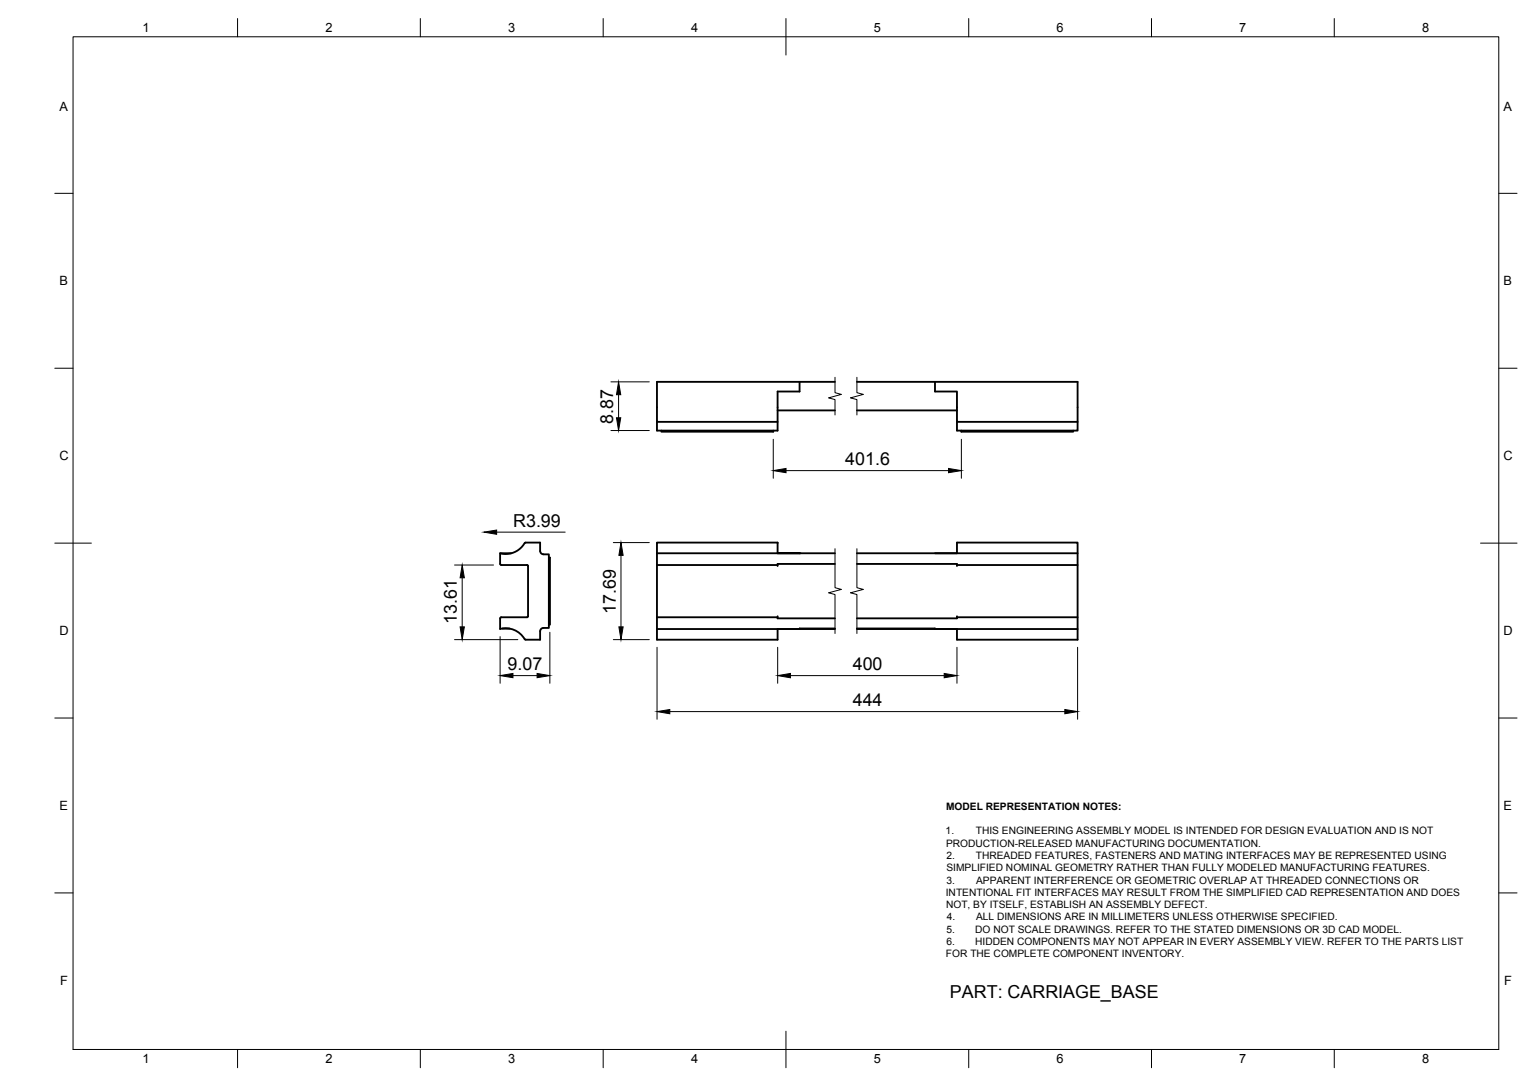
ISO-10303-21;
HEADER;
/* Generated by software containing ST-Developer
 * from STEP Tools, Inc. (www.steptools.com) 
 */

FILE_DESCRIPTION(
/* description */ (''),
/* implementation_level */ '2;1');

FILE_NAME(
/* name */ 'Carriage_Base.step',
/* time_stamp */ '2026-10-05T11:01:41-07:00',
/* author */ (''),
/* organization */ (''),
/* preprocessor_version */ 'ST-DEVELOPER v20.2',
/* originating_system */ 'Autodesk Translation Framework v15.15.0.0',
/* authorisation */ '');

FILE_SCHEMA (('AUTOMOTIVE_DESIGN { 1 0 10303 214 3 1 1 }'));
ENDSEC;

DATA;
#10=MECHANICAL_DESIGN_GEOMETRIC_PRESENTATION_REPRESENTATION('',(#2143),#215609);
#216=FACE_BOUND('',#5119,.T.);
#217=FACE_BOUND('',#5154,.T.);
#2125=SHAPE_REPRESENTATION_RELATIONSHIP('SRR','None',#215650,#2134);
#2134=ADVANCED_BREP_SHAPE_REPRESENTATION('',(#2152),#215606);
#2143=STYLED_ITEM('',(#215698),#2152);
#2152=MANIFOLD_SOLID_BREP('Body1',#28086);
#2632=CYLINDRICAL_SURFACE('',#29448,0.190999999999998);
#2633=CYLINDRICAL_SURFACE('',#29461,0.191);
#2634=CYLINDRICAL_SURFACE('',#29467,3.9858295958384);
#2635=CYLINDRICAL_SURFACE('',#29468,3.9858295958384);
#2636=CYLINDRICAL_SURFACE('',#29480,0.190999999999999);
#2637=CYLINDRICAL_SURFACE('',#29482,0.191);
#2638=CYLINDRICAL_SURFACE('',#29483,0.590999999999999);
#2639=CYLINDRICAL_SURFACE('',#29484,0.590999999999999);
#2640=CYLINDRICAL_SURFACE('',#29485,0.191000000000001);
#2641=CYLINDRICAL_SURFACE('',#29487,0.190999999999999);
#2642=CYLINDRICAL_SURFACE('',#29504,0.190999999999998);
#2643=CYLINDRICAL_SURFACE('',#29518,0.191);
#2644=CYLINDRICAL_SURFACE('',#29524,3.9858295958384);
#2645=CYLINDRICAL_SURFACE('',#29525,3.9858295958384);
#2646=CYLINDRICAL_SURFACE('',#29542,0.190999999999999);
#2647=CYLINDRICAL_SURFACE('',#29544,0.191);
#2648=CYLINDRICAL_SURFACE('',#29545,0.590999999999999);
#2649=CYLINDRICAL_SURFACE('',#29546,0.590999999999999);
#2650=CYLINDRICAL_SURFACE('',#29547,0.191000000000001);
#2651=CYLINDRICAL_SURFACE('',#29549,0.190999999999999);
#3752=FACE_OUTER_BOUND('',#5108,.T.);
#3753=FACE_OUTER_BOUND('',#5109,.T.);
#3754=FACE_OUTER_BOUND('',#5110,.T.);
#3755=FACE_OUTER_BOUND('',#5111,.T.);
#3756=FACE_OUTER_BOUND('',#5112,.T.);
#3757=FACE_OUTER_BOUND('',#5113,.T.);
#3758=FACE_OUTER_BOUND('',#5114,.T.);
#3759=FACE_OUTER_BOUND('',#5115,.T.);
#3760=FACE_OUTER_BOUND('',#5116,.T.);
#3761=FACE_OUTER_BOUND('',#5117,.T.);
#3762=FACE_OUTER_BOUND('',#5118,.T.);
#3763=FACE_OUTER_BOUND('',#5120,.T.);
#3764=FACE_OUTER_BOUND('',#5121,.T.);
#3765=FACE_OUTER_BOUND('',#5122,.T.);
#3766=FACE_OUTER_BOUND('',#5123,.T.);
#3767=FACE_OUTER_BOUND('',#5124,.T.);
#3768=FACE_OUTER_BOUND('',#5125,.T.);
#3769=FACE_OUTER_BOUND('',#5126,.T.);
#3770=FACE_OUTER_BOUND('',#5127,.T.);
#3771=FACE_OUTER_BOUND('',#5128,.T.);
#3772=FACE_OUTER_BOUND('',#5129,.T.);
#3773=FACE_OUTER_BOUND('',#5130,.T.);
#3774=FACE_OUTER_BOUND('',#5131,.T.);
#3775=FACE_OUTER_BOUND('',#5132,.T.);
#3776=FACE_OUTER_BOUND('',#5133,.T.);
#3777=FACE_OUTER_BOUND('',#5134,.T.);
#3778=FACE_OUTER_BOUND('',#5135,.T.);
#3779=FACE_OUTER_BOUND('',#5136,.T.);
#3780=FACE_OUTER_BOUND('',#5137,.T.);
#3781=FACE_OUTER_BOUND('',#5138,.T.);
#3782=FACE_OUTER_BOUND('',#5139,.T.);
#3783=FACE_OUTER_BOUND('',#5140,.T.);
#3784=FACE_OUTER_BOUND('',#5141,.T.);
#3785=FACE_OUTER_BOUND('',#5142,.T.);
#3786=FACE_OUTER_BOUND('',#5143,.T.);
#3787=FACE_OUTER_BOUND('',#5144,.T.);
#3788=FACE_OUTER_BOUND('',#5145,.T.);
#3789=FACE_OUTER_BOUND('',#5146,.T.);
#3790=FACE_OUTER_BOUND('',#5147,.T.);
#3791=FACE_OUTER_BOUND('',#5148,.T.);
#3792=FACE_OUTER_BOUND('',#5149,.T.);
#3793=FACE_OUTER_BOUND('',#5150,.T.);
#3794=FACE_OUTER_BOUND('',#5151,.T.);
#3795=FACE_OUTER_BOUND('',#5152,.T.);
#3796=FACE_OUTER_BOUND('',#5153,.T.);
#3797=FACE_OUTER_BOUND('',#5155,.T.);
#3798=FACE_OUTER_BOUND('',#5156,.T.);
#3799=FACE_OUTER_BOUND('',#5157,.T.);
#3800=FACE_OUTER_BOUND('',#5158,.T.);
#3801=FACE_OUTER_BOUND('',#5159,.T.);
#3802=FACE_OUTER_BOUND('',#5160,.T.);
#3803=FACE_OUTER_BOUND('',#5161,.T.);
#3804=FACE_OUTER_BOUND('',#5162,.T.);
#3805=FACE_OUTER_BOUND('',#5163,.T.);
#3806=FACE_OUTER_BOUND('',#5164,.T.);
#3807=FACE_OUTER_BOUND('',#5165,.T.);
#3808=FACE_OUTER_BOUND('',#5166,.T.);
#3809=FACE_OUTER_BOUND('',#5167,.T.);
#3810=FACE_OUTER_BOUND('',#5168,.T.);
#3811=FACE_OUTER_BOUND('',#5169,.T.);
#3812=FACE_OUTER_BOUND('',#5170,.T.);
#3813=FACE_OUTER_BOUND('',#5171,.T.);
#3814=FACE_OUTER_BOUND('',#5172,.T.);
#3815=FACE_OUTER_BOUND('',#5173,.T.);
#3816=FACE_OUTER_BOUND('',#5174,.T.);
#3817=FACE_OUTER_BOUND('',#5175,.T.);
#3818=FACE_OUTER_BOUND('',#5176,.T.);
#3819=FACE_OUTER_BOUND('',#5177,.T.);
#3820=FACE_OUTER_BOUND('',#5178,.T.);
#3821=FACE_OUTER_BOUND('',#5179,.T.);
#5108=EDGE_LOOP('',(#22607,#22608,#22609));
#5109=EDGE_LOOP('',(#22610,#22611,#22612));
#5110=EDGE_LOOP('',(#22613,#22614));
#5111=EDGE_LOOP('',(#22615,#22616,#22617,#22618));
#5112=EDGE_LOOP('',(#22619,#22620,#22621,#22622,#22623,#22624,#22625,#22626,
#22627,#22628,#22629,#22630,#22631,#22632,#22633,#22634));
#5113=EDGE_LOOP('',(#22635,#22636,#22637,#22638));
#5114=EDGE_LOOP('',(#22639,#22640,#22641,#22642));
#5115=EDGE_LOOP('',(#22643,#22644,#22645,#22646,#22647,#22648,#22649,#22650,
#22651,#22652,#22653,#22654,#22655,#22656,#22657,#22658,#22659,#22660,#22661,
#22662,#22663,#22664));
#5116=EDGE_LOOP('',(#22665,#22666,#22667,#22668));
#5117=EDGE_LOOP('',(#22669,#22670,#22671,#22672));
#5118=EDGE_LOOP('',(#22673,#22674,#22675,#22676));
#5119=EDGE_LOOP('',(#22677,#22678,#22679,#22680));
#5120=EDGE_LOOP('',(#22681,#22682,#22683,#22684));
#5121=EDGE_LOOP('',(#22685,#22686,#22687,#22688));
#5122=EDGE_LOOP('',(#22689,#22690,#22691,#22692));
#5123=EDGE_LOOP('',(#22693,#22694,#22695,#22696,#22697,#22698));
#5124=EDGE_LOOP('',(#22699,#22700,#22701,#22702,#22703,#22704,#22705));
#5125=EDGE_LOOP('',(#22706,#22707,#22708,#22709));
#5126=EDGE_LOOP('',(#22710,#22711,#22712,#22713));
#5127=EDGE_LOOP('',(#22714,#22715,#22716,#22717));
#5128=EDGE_LOOP('',(#22718,#22719,#22720,#22721));
#5129=EDGE_LOOP('',(#22722,#22723,#22724,#22725));
#5130=EDGE_LOOP('',(#22726,#22727,#22728,#22729,#22730));
#5131=EDGE_LOOP('',(#22731,#22732,#22733,#22734,#22735));
#5132=EDGE_LOOP('',(#22736,#22737,#22738,#22739));
#5133=EDGE_LOOP('',(#22740,#22741,#22742,#22743));
#5134=EDGE_LOOP('',(#22744,#22745,#22746,#22747));
#5135=EDGE_LOOP('',(#22748,#22749,#22750,#22751));
#5136=EDGE_LOOP('',(#22752,#22753,#22754,#22755));
#5137=EDGE_LOOP('',(#22756,#22757,#22758,#22759));
#5138=EDGE_LOOP('',(#22760,#22761,#22762,#22763));
#5139=EDGE_LOOP('',(#22764,#22765,#22766,#22767));
#5140=EDGE_LOOP('',(#22768,#22769,#22770));
#5141=EDGE_LOOP('',(#22771,#22772,#22773));
#5142=EDGE_LOOP('',(#22774,#22775));
#5143=EDGE_LOOP('',(#22776,#22777,#22778,#22779,#22780,#22781,#22782,#22783));
#5144=EDGE_LOOP('',(#22784,#22785,#22786,#22787));
#5145=EDGE_LOOP('',(#22788,#22789,#22790,#22791,#22792,#22793,#22794,#22795,
#22796,#22797,#22798,#22799,#22800,#22801,#22802,#22803));
#5146=EDGE_LOOP('',(#22804,#22805,#22806,#22807,#22808,#22809,#22810,#22811,
#22812,#22813));
#5147=EDGE_LOOP('',(#22814,#22815,#22816,#22817));
#5148=EDGE_LOOP('',(#22818,#22819,#22820,#22821));
#5149=EDGE_LOOP('',(#22822,#22823,#22824,#22825,#22826,#22827,#22828,#22829,
#22830,#22831,#22832,#22833,#22834,#22835,#22836,#22837,#22838,#22839,#22840,
#22841,#22842,#22843));
#5150=EDGE_LOOP('',(#22844,#22845,#22846,#22847,#22848,#22849,#22850,#22851,
#22852,#22853));
#5151=EDGE_LOOP('',(#22854,#22855,#22856,#22857));
#5152=EDGE_LOOP('',(#22858,#22859,#22860,#22861));
#5153=EDGE_LOOP('',(#22862,#22863,#22864,#22865));
#5154=EDGE_LOOP('',(#22866,#22867,#22868,#22869));
#5155=EDGE_LOOP('',(#22870,#22871,#22872,#22873));
#5156=EDGE_LOOP('',(#22874,#22875,#22876,#22877));
#5157=EDGE_LOOP('',(#22878,#22879,#22880,#22881));
#5158=EDGE_LOOP('',(#22882,#22883,#22884,#22885,#22886,#22887));
#5159=EDGE_LOOP('',(#22888,#22889,#22890,#22891,#22892,#22893,#22894));
#5160=EDGE_LOOP('',(#22895,#22896,#22897,#22898));
#5161=EDGE_LOOP('',(#22899,#22900,#22901,#22902));
#5162=EDGE_LOOP('',(#22903,#22904,#22905,#22906));
#5163=EDGE_LOOP('',(#22907,#22908,#22909,#22910));
#5164=EDGE_LOOP('',(#22911,#22912,#22913,#22914));
#5165=EDGE_LOOP('',(#22915,#22916,#22917,#22918));
#5166=EDGE_LOOP('',(#22919,#22920,#22921,#22922));
#5167=EDGE_LOOP('',(#22923,#22924,#22925,#22926));
#5168=EDGE_LOOP('',(#22927,#22928,#22929,#22930,#22931));
#5169=EDGE_LOOP('',(#22932,#22933,#22934,#22935,#22936));
#5170=EDGE_LOOP('',(#22937,#22938,#22939,#22940,#22941,#22942,#22943,#22944,
#22945,#22946));
#5171=EDGE_LOOP('',(#22947,#22948,#22949,#22950,#22951,#22952,#22953,#22954,
#22955,#22956,#22957,#22958));
#5172=EDGE_LOOP('',(#22959,#22960,#22961,#22962));
#5173=EDGE_LOOP('',(#22963,#22964,#22965,#22966));
#5174=EDGE_LOOP('',(#22967,#22968,#22969,#22970));
#5175=EDGE_LOOP('',(#22971,#22972,#22973,#22974));
#5176=EDGE_LOOP('',(#22975,#22976,#22977,#22978));
#5177=EDGE_LOOP('',(#22979,#22980,#22981,#22982));
#5178=EDGE_LOOP('',(#22983,#22984,#22985,#22986));
#5179=EDGE_LOOP('',(#22987,#22988,#22989,#22990));
#6088=CIRCLE('',#29435,3.9858295958384);
#6089=CIRCLE('',#29437,3.9858295958384);
#6090=CIRCLE('',#29439,3.9858295958384);
#6091=CIRCLE('',#29442,3.9858295958384);
#6092=CIRCLE('',#29443,3.9858295958384);
#6093=CIRCLE('',#29444,0.191);
#6094=CIRCLE('',#29445,0.590999999999999);
#6095=CIRCLE('',#29446,0.590999999999999);
#6096=CIRCLE('',#29447,0.190999999999998);
#6097=CIRCLE('',#29449,0.190999999999998);
#6098=CIRCLE('',#29452,0.590999999999999);
#6099=CIRCLE('',#29453,0.590999999999999);
#6100=CIRCLE('',#29454,0.191);
#6101=CIRCLE('',#29455,3.9858295958384);
#6102=CIRCLE('',#29456,0.191000000000001);
#6103=CIRCLE('',#29457,0.190999999999999);
#6104=CIRCLE('',#29458,0.190999999999999);
#6105=CIRCLE('',#29459,0.191);
#6106=CIRCLE('',#29460,3.9858295958384);
#6107=CIRCLE('',#29475,0.191);
#6108=CIRCLE('',#29476,0.190999999999999);
#6109=CIRCLE('',#29478,0.190999999999999);
#6110=CIRCLE('',#29479,0.191000000000001);
#6111=CIRCLE('',#29489,3.9858295958384);
#6112=CIRCLE('',#29491,3.9858295958384);
#6113=CIRCLE('',#29493,3.9858295958384);
#6114=CIRCLE('',#29497,3.9858295958384);
#6115=CIRCLE('',#29498,0.190999999999998);
#6116=CIRCLE('',#29499,0.590999999999999);
#6117=CIRCLE('',#29500,0.590999999999999);
#6118=CIRCLE('',#29501,0.191);
#6119=CIRCLE('',#29502,3.9858295958384);
#6120=CIRCLE('',#29505,0.190999999999998);
#6121=CIRCLE('',#29508,3.9858295958384);
#6122=CIRCLE('',#29509,0.191);
#6123=CIRCLE('',#29510,0.190999999999999);
#6124=CIRCLE('',#29511,0.190999999999999);
#6125=CIRCLE('',#29512,0.191000000000001);
#6126=CIRCLE('',#29513,3.9858295958384);
#6127=CIRCLE('',#29514,0.191);
#6128=CIRCLE('',#29515,0.590999999999999);
#6129=CIRCLE('',#29516,0.590999999999999);
#6130=CIRCLE('',#29535,0.190999999999999);
#6131=CIRCLE('',#29536,0.191);
#6132=CIRCLE('',#29538,0.191000000000001);
#6133=CIRCLE('',#29539,0.190999999999999);
#7371=LINE('',#127456,#9216);
#7372=LINE('',#127458,#9217);
#7373=LINE('',#127463,#9218);
#7374=LINE('',#127466,#9219);
#7375=LINE('',#127470,#9220);
#7376=LINE('',#127474,#9221);
#7377=LINE('',#127476,#9222);
#7378=LINE('',#127478,#9223);
#7379=LINE('',#127479,#9224);
#7380=LINE('',#127485,#9225);
#7381=LINE('',#127487,#9226);
#7382=LINE('',#127489,#9227);
#7383=LINE('',#127494,#9228);
#7384=LINE('',#127498,#9229);
#7385=LINE('',#127500,#9230);
#7386=LINE('',#127502,#9231);
#7387=LINE('',#127506,#9232);
#7388=LINE('',#127508,#9233);
#7389=LINE('',#127514,#9234);
#7390=LINE('',#127515,#9235);
#7391=LINE('',#127518,#9236);
#7392=LINE('',#127519,#9237);
#7393=LINE('',#127522,#9238);
#7394=LINE('',#127526,#9239);
#7395=LINE('',#127528,#9240);
#7396=LINE('',#127530,#9241);
#7397=LINE('',#127533,#9242);
#7398=LINE('',#127539,#9243);
#7399=LINE('',#127543,#9244);
#7400=LINE('',#127547,#9245);
#7401=LINE('',#127551,#9246);
#7402=LINE('',#127555,#9247);
#7403=LINE('',#127558,#9248);
#7404=LINE('',#127560,#9249);
#7405=LINE('',#127562,#9250);
#7406=LINE('',#127563,#9251);
#7407=LINE('',#127566,#9252);
#7408=LINE('',#127568,#9253);
#7409=LINE('',#127570,#9254);
#7410=LINE('',#127571,#9255);
#7411=LINE('',#127573,#9256);
#7412=LINE('',#127575,#9257);
#7413=LINE('',#127577,#9258);
#7414=LINE('',#127579,#9259);
#7415=LINE('',#127580,#9260);
#7416=LINE('',#127582,#9261);
#7417=LINE('',#127583,#9262);
#7418=LINE('',#127586,#9263);
#7419=LINE('',#127588,#9264);
#7420=LINE('',#127589,#9265);
#7421=LINE('',#127592,#9266);
#7422=LINE('',#127593,#9267);
#7423=LINE('',#127596,#9268);
#7424=LINE('',#127597,#9269);
#7425=LINE('',#127599,#9270);
#7426=LINE('',#127604,#9271);
#7427=LINE('',#127608,#9272);
#7428=LINE('',#127611,#9273);
#7429=LINE('',#127615,#9274);
#7430=LINE('',#127617,#9275);
#7431=LINE('',#127621,#9276);
#7432=LINE('',#127624,#9277);
#7433=LINE('',#127625,#9278);
#7434=LINE('',#127627,#9279);
#7435=LINE('',#127629,#9280);
#7436=LINE('',#127633,#9281);
#7437=LINE('',#127634,#9282);
#7438=LINE('',#127636,#9283);
#7439=LINE('',#127638,#9284);
#7440=LINE('',#127642,#9285);
#7441=LINE('',#127645,#9286);
#7442=LINE('',#127649,#9287);
#7443=LINE('',#127651,#9288);
#7444=LINE('',#127656,#9289);
#7445=LINE('',#127659,#9290);
#7446=LINE('',#127661,#9291);
#7447=LINE('',#127662,#9292);
#7448=LINE('',#127663,#9293);
#7449=LINE('',#127667,#9294);
#7450=LINE('',#127669,#9295);
#7451=LINE('',#127671,#9296);
#7452=LINE('',#127672,#9297);
#7453=LINE('',#127679,#9298);
#7454=LINE('',#127681,#9299);
#7455=LINE('',#127685,#9300);
#7456=LINE('',#127687,#9301);
#7457=LINE('',#127689,#9302);
#7458=LINE('',#127692,#9303);
#7459=LINE('',#127698,#9304);
#7460=LINE('',#127699,#9305);
#7461=LINE('',#127701,#9306);
#7462=LINE('',#127702,#9307);
#7463=LINE('',#127703,#9308);
#7464=LINE('',#127708,#9309);
#7465=LINE('',#127709,#9310);
#7466=LINE('',#127712,#9311);
#7467=LINE('',#127713,#9312);
#7468=LINE('',#127718,#9313);
#7469=LINE('',#127722,#9314);
#7470=LINE('',#127726,#9315);
#7471=LINE('',#127730,#9316);
#7472=LINE('',#127734,#9317);
#7473=LINE('',#127739,#9318);
#7474=LINE('',#127743,#9319);
#7475=LINE('',#127745,#9320);
#7476=LINE('',#127747,#9321);
#7477=LINE('',#127750,#9322);
#7478=LINE('',#127753,#9323);
#7479=LINE('',#127754,#9324);
#7480=LINE('',#127755,#9325);
#7481=LINE('',#127757,#9326);
#7482=LINE('',#127759,#9327);
#7483=LINE('',#127761,#9328);
#7484=LINE('',#127762,#9329);
#7485=LINE('',#127765,#9330);
#7486=LINE('',#127767,#9331);
#7487=LINE('',#127769,#9332);
#7488=LINE('',#127770,#9333);
#7489=LINE('',#127772,#9334);
#7490=LINE('',#127774,#9335);
#7491=LINE('',#127776,#9336);
#7492=LINE('',#127779,#9337);
#7493=LINE('',#127782,#9338);
#7494=LINE('',#127784,#9339);
#7495=LINE('',#127785,#9340);
#7496=LINE('',#127788,#9341);
#7497=LINE('',#127789,#9342);
#7498=LINE('',#127792,#9343);
#7499=LINE('',#127793,#9344);
#7500=LINE('',#127795,#9345);
#7501=LINE('',#127800,#9346);
#7502=LINE('',#127801,#9347);
#7503=LINE('',#127805,#9348);
#7504=LINE('',#127806,#9349);
#7505=LINE('',#127807,#9350);
#7506=LINE('',#127810,#9351);
#7507=LINE('',#127814,#9352);
#7508=LINE('',#127820,#9353);
#7509=LINE('',#127823,#9354);
#7510=LINE('',#127825,#9355);
#7511=LINE('',#127827,#9356);
#7512=LINE('',#127828,#9357);
#7513=LINE('',#127830,#9358);
#7514=LINE('',#127832,#9359);
#7515=LINE('',#127837,#9360);
#7516=LINE('',#127839,#9361);
#9216=VECTOR('',#33753,10.);
#9217=VECTOR('',#33754,10.);
#9218=VECTOR('',#33759,10.);
#9219=VECTOR('',#33762,10.);
#9220=VECTOR('',#33767,10.);
#9221=VECTOR('',#33770,10.);
#9222=VECTOR('',#33771,10.);
#9223=VECTOR('',#33772,10.);
#9224=VECTOR('',#33773,10.);
#9225=VECTOR('',#33778,10.);
#9226=VECTOR('',#33779,10.);
#9227=VECTOR('',#33780,10.);
#9228=VECTOR('',#33785,10.);
#9229=VECTOR('',#33788,10.);
#9230=VECTOR('',#33789,10.);
#9231=VECTOR('',#33790,10.);
#9232=VECTOR('',#33793,10.);
#9233=VECTOR('',#33794,10.);
#9234=VECTOR('',#33801,10.);
#9235=VECTOR('',#33802,10.);
#9236=VECTOR('',#33805,10.);
#9237=VECTOR('',#33806,10.);
#9238=VECTOR('',#33809,10.);
#9239=VECTOR('',#33812,10.);
#9240=VECTOR('',#33813,10.);
#9241=VECTOR('',#33814,10.);
#9242=VECTOR('',#33817,10.);
#9243=VECTOR('',#33822,10.);
#9244=VECTOR('',#33825,10.);
#9245=VECTOR('',#33828,10.);
#9246=VECTOR('',#33831,10.);
#9247=VECTOR('',#33834,10.);
#9248=VECTOR('',#33839,10.);
#9249=VECTOR('',#33842,10.);
#9250=VECTOR('',#33845,10.);
#9251=VECTOR('',#33846,10.);
#9252=VECTOR('',#33847,10.);
#9253=VECTOR('',#33848,10.);
#9254=VECTOR('',#33849,10.);
#9255=VECTOR('',#33850,10.);
#9256=VECTOR('',#33853,10.);
#9257=VECTOR('',#33856,10.);
#9258=VECTOR('',#33859,10.);
#9259=VECTOR('',#33862,10.);
#9260=VECTOR('',#33863,10.);
#9261=VECTOR('',#33866,10.);
#9262=VECTOR('',#33867,10.);
#9263=VECTOR('',#33870,10.);
#9264=VECTOR('',#33871,10.);
#9265=VECTOR('',#33872,10.);
#9266=VECTOR('',#33875,10.);
#9267=VECTOR('',#33876,10.);
#9268=VECTOR('',#33879,10.);
#9269=VECTOR('',#33880,10.);
#9270=VECTOR('',#33883,10.);
#9271=VECTOR('',#33888,10.);
#9272=VECTOR('',#33891,10.);
#9273=VECTOR('',#33894,10.);
#9274=VECTOR('',#33897,10.);
#9275=VECTOR('',#33898,10.);
#9276=VECTOR('',#33901,10.);
#9277=VECTOR('',#33906,10.);
#9278=VECTOR('',#33907,10.);
#9279=VECTOR('',#33910,10.);
#9280=VECTOR('',#33913,10.);
#9281=VECTOR('',#33920,10.);
#9282=VECTOR('',#33921,10.);
#9283=VECTOR('',#33924,10.);
#9284=VECTOR('',#33927,10.);
#9285=VECTOR('',#33930,10.);
#9286=VECTOR('',#33933,10.);
#9287=VECTOR('',#33936,10.);
#9288=VECTOR('',#33937,10.);
#9289=VECTOR('',#33944,10.);
#9290=VECTOR('',#33947,10.);
#9291=VECTOR('',#33948,10.);
#9292=VECTOR('',#33949,10.);
#9293=VECTOR('',#33950,10.);
#9294=VECTOR('',#33953,10.);
#9295=VECTOR('',#33954,10.);
#9296=VECTOR('',#33955,10.);
#9297=VECTOR('',#33956,10.);
#9298=VECTOR('',#33963,10.);
#9299=VECTOR('',#33964,10.);
#9300=VECTOR('',#33967,10.);
#9301=VECTOR('',#33968,10.);
#9302=VECTOR('',#33969,10.);
#9303=VECTOR('',#33972,10.);
#9304=VECTOR('',#33977,10.);
#9305=VECTOR('',#33978,10.);
#9306=VECTOR('',#33981,10.);
#9307=VECTOR('',#33982,10.);
#9308=VECTOR('',#33983,10.);
#9309=VECTOR('',#33988,10.);
#9310=VECTOR('',#33989,10.);
#9311=VECTOR('',#33992,10.);
#9312=VECTOR('',#33993,10.);
#9313=VECTOR('',#33998,10.);
#9314=VECTOR('',#34001,10.);
#9315=VECTOR('',#34004,10.);
#9316=VECTOR('',#34007,10.);
#9317=VECTOR('',#34010,10.);
#9318=VECTOR('',#34015,10.);
#9319=VECTOR('',#34018,10.);
#9320=VECTOR('',#34019,10.);
#9321=VECTOR('',#34020,10.);
#9322=VECTOR('',#34023,10.);
#9323=VECTOR('',#34026,10.);
#9324=VECTOR('',#34027,10.);
#9325=VECTOR('',#34028,10.);
#9326=VECTOR('',#34031,10.);
#9327=VECTOR('',#34034,10.);
#9328=VECTOR('',#34037,10.);
#9329=VECTOR('',#34038,10.);
#9330=VECTOR('',#34039,10.);
#9331=VECTOR('',#34040,10.);
#9332=VECTOR('',#34041,10.);
#9333=VECTOR('',#34042,10.);
#9334=VECTOR('',#34045,10.);
#9335=VECTOR('',#34048,10.);
#9336=VECTOR('',#34051,10.);
#9337=VECTOR('',#34056,10.);
#9338=VECTOR('',#34059,10.);
#9339=VECTOR('',#34060,10.);
#9340=VECTOR('',#34061,10.);
#9341=VECTOR('',#34064,10.);
#9342=VECTOR('',#34065,10.);
#9343=VECTOR('',#34068,10.);
#9344=VECTOR('',#34069,10.);
#9345=VECTOR('',#34072,10.);
#9346=VECTOR('',#34079,10.);
#9347=VECTOR('',#34080,10.);
#9348=VECTOR('',#34083,10.);
#9349=VECTOR('',#34084,10.);
#9350=VECTOR('',#34085,10.);
#9351=VECTOR('',#34088,10.);
#9352=VECTOR('',#34091,10.);
#9353=VECTOR('',#34098,10.);
#9354=VECTOR('',#34101,10.);
#9355=VECTOR('',#34104,10.);
#9356=VECTOR('',#34107,10.);
#9357=VECTOR('',#34108,10.);
#9358=VECTOR('',#34111,10.);
#9359=VECTOR('',#34114,10.);
#9360=VECTOR('',#34123,10.);
#9361=VECTOR('',#34126,10.);
#11760=VERTEX_POINT('',#127454);
#11761=VERTEX_POINT('',#127455);
#11762=VERTEX_POINT('',#127457);
#11763=VERTEX_POINT('',#127461);
#11764=VERTEX_POINT('',#127462);
#11765=VERTEX_POINT('',#127464);
#11766=VERTEX_POINT('',#127468);
#11767=VERTEX_POINT('',#127472);
#11768=VERTEX_POINT('',#127473);
#11769=VERTEX_POINT('',#127475);
#11770=VERTEX_POINT('',#127477);
#11771=VERTEX_POINT('',#127481);
#11772=VERTEX_POINT('',#127482);
#11773=VERTEX_POINT('',#127484);
#11774=VERTEX_POINT('',#127486);
#11775=VERTEX_POINT('',#127488);
#11776=VERTEX_POINT('',#127490);
#11777=VERTEX_POINT('',#127493);
#11778=VERTEX_POINT('',#127495);
#11779=VERTEX_POINT('',#127497);
#11780=VERTEX_POINT('',#127499);
#11781=VERTEX_POINT('',#127501);
#11782=VERTEX_POINT('',#127503);
#11783=VERTEX_POINT('',#127505);
#11784=VERTEX_POINT('',#127507);
#11785=VERTEX_POINT('',#127511);
#11786=VERTEX_POINT('',#127512);
#11787=VERTEX_POINT('',#127517);
#11788=VERTEX_POINT('',#127521);
#11789=VERTEX_POINT('',#127523);
#11790=VERTEX_POINT('',#127525);
#11791=VERTEX_POINT('',#127527);
#11792=VERTEX_POINT('',#127529);
#11793=VERTEX_POINT('',#127531);
#11794=VERTEX_POINT('',#127534);
#11795=VERTEX_POINT('',#127536);
#11796=VERTEX_POINT('',#127538);
#11797=VERTEX_POINT('',#127540);
#11798=VERTEX_POINT('',#127542);
#11799=VERTEX_POINT('',#127544);
#11800=VERTEX_POINT('',#127546);
#11801=VERTEX_POINT('',#127548);
#11802=VERTEX_POINT('',#127550);
#11803=VERTEX_POINT('',#127552);
#11804=VERTEX_POINT('',#127554);
#11805=VERTEX_POINT('',#127564);
#11806=VERTEX_POINT('',#127565);
#11807=VERTEX_POINT('',#127567);
#11808=VERTEX_POINT('',#127569);
#11809=VERTEX_POINT('',#127585);
#11810=VERTEX_POINT('',#127587);
#11811=VERTEX_POINT('',#127591);
#11812=VERTEX_POINT('',#127595);
#11813=VERTEX_POINT('',#127602);
#11814=VERTEX_POINT('',#127603);
#11815=VERTEX_POINT('',#127605);
#11816=VERTEX_POINT('',#127607);
#11817=VERTEX_POINT('',#127609);
#11818=VERTEX_POINT('',#127613);
#11819=VERTEX_POINT('',#127614);
#11820=VERTEX_POINT('',#127616);
#11821=VERTEX_POINT('',#127618);
#11822=VERTEX_POINT('',#127620);
#11823=VERTEX_POINT('',#127640);
#11824=VERTEX_POINT('',#127641);
#11825=VERTEX_POINT('',#127643);
#11826=VERTEX_POINT('',#127647);
#11827=VERTEX_POINT('',#127648);
#11828=VERTEX_POINT('',#127650);
#11829=VERTEX_POINT('',#127654);
#11830=VERTEX_POINT('',#127658);
#11831=VERTEX_POINT('',#127660);
#11832=VERTEX_POINT('',#127665);
#11833=VERTEX_POINT('',#127666);
#11834=VERTEX_POINT('',#127668);
#11835=VERTEX_POINT('',#127670);
#11836=VERTEX_POINT('',#127674);
#11837=VERTEX_POINT('',#127676);
#11838=VERTEX_POINT('',#127678);
#11839=VERTEX_POINT('',#127680);
#11840=VERTEX_POINT('',#127682);
#11841=VERTEX_POINT('',#127684);
#11842=VERTEX_POINT('',#127686);
#11843=VERTEX_POINT('',#127688);
#11844=VERTEX_POINT('',#127690);
#11845=VERTEX_POINT('',#127693);
#11846=VERTEX_POINT('',#127695);
#11847=VERTEX_POINT('',#127697);
#11848=VERTEX_POINT('',#127705);
#11849=VERTEX_POINT('',#127706);
#11850=VERTEX_POINT('',#127711);
#11851=VERTEX_POINT('',#127715);
#11852=VERTEX_POINT('',#127717);
#11853=VERTEX_POINT('',#127719);
#11854=VERTEX_POINT('',#127721);
#11855=VERTEX_POINT('',#127723);
#11856=VERTEX_POINT('',#127725);
#11857=VERTEX_POINT('',#127727);
#11858=VERTEX_POINT('',#127729);
#11859=VERTEX_POINT('',#127731);
#11860=VERTEX_POINT('',#127733);
#11861=VERTEX_POINT('',#127735);
#11862=VERTEX_POINT('',#127738);
#11863=VERTEX_POINT('',#127740);
#11864=VERTEX_POINT('',#127742);
#11865=VERTEX_POINT('',#127744);
#11866=VERTEX_POINT('',#127746);
#11867=VERTEX_POINT('',#127748);
#11868=VERTEX_POINT('',#127752);
#11869=VERTEX_POINT('',#127763);
#11870=VERTEX_POINT('',#127764);
#11871=VERTEX_POINT('',#127766);
#11872=VERTEX_POINT('',#127768);
#11873=VERTEX_POINT('',#127781);
#11874=VERTEX_POINT('',#127783);
#11875=VERTEX_POINT('',#127787);
#11876=VERTEX_POINT('',#127791);
#11877=VERTEX_POINT('',#127799);
#11878=VERTEX_POINT('',#127803);
#11879=VERTEX_POINT('',#127804);
#11880=VERTEX_POINT('',#127809);
#11881=VERTEX_POINT('',#127811);
#11882=VERTEX_POINT('',#127813);
#11883=VERTEX_POINT('',#127817);
#11884=VERTEX_POINT('',#127819);
#11885=VERTEX_POINT('',#127821);
#15665=EDGE_CURVE('',#11760,#11761,#7371,.T.);
#15666=EDGE_CURVE('',#11761,#11762,#7372,.F.);
#15667=EDGE_CURVE('',#11762,#11760,#6088,.T.);
#15668=EDGE_CURVE('',#11763,#11764,#7373,.T.);
#15669=EDGE_CURVE('',#11764,#11765,#6089,.T.);
#15670=EDGE_CURVE('',#11765,#11763,#7374,.T.);
#15671=EDGE_CURVE('',#11760,#11766,#6090,.T.);
#15672=EDGE_CURVE('',#11766,#11760,#7375,.T.);
#15673=EDGE_CURVE('',#11767,#11768,#7376,.T.);
#15674=EDGE_CURVE('',#11768,#11769,#7377,.T.);
#15675=EDGE_CURVE('',#11769,#11770,#7378,.F.);
#15676=EDGE_CURVE('',#11767,#11770,#7379,.T.);
#15677=EDGE_CURVE('',#11771,#11772,#6091,.T.);
#15678=EDGE_CURVE('',#11773,#11771,#7380,.T.);
#15679=EDGE_CURVE('',#11774,#11773,#7381,.T.);
#15680=EDGE_CURVE('',#11775,#11774,#7382,.T.);
#15681=EDGE_CURVE('',#11776,#11775,#6092,.T.);
#15682=EDGE_CURVE('',#11767,#11776,#6093,.T.);
#15683=EDGE_CURVE('',#11770,#11777,#7383,.T.);
#15684=EDGE_CURVE('',#11777,#11778,#6094,.T.);
#15685=EDGE_CURVE('',#11778,#11779,#7384,.T.);
#15686=EDGE_CURVE('',#11780,#11779,#7385,.F.);
#15687=EDGE_CURVE('',#11781,#11780,#7386,.F.);
#15688=EDGE_CURVE('',#11781,#11782,#6095,.T.);
#15689=EDGE_CURVE('',#11783,#11782,#7387,.F.);
#15690=EDGE_CURVE('',#11784,#11783,#7388,.F.);
#15691=EDGE_CURVE('',#11772,#11784,#6096,.T.);
#15692=EDGE_CURVE('',#11785,#11786,#6097,.T.);
#15693=EDGE_CURVE('',#11785,#11772,#7389,.T.);
#15694=EDGE_CURVE('',#11784,#11786,#7390,.T.);
#15695=EDGE_CURVE('',#11787,#11783,#7391,.F.);
#15696=EDGE_CURVE('',#11787,#11786,#7392,.T.);
#15697=EDGE_CURVE('',#11788,#11787,#7393,.T.);
#15698=EDGE_CURVE('',#11789,#11788,#6098,.T.);
#15699=EDGE_CURVE('',#11790,#11789,#7394,.T.);
#15700=EDGE_CURVE('',#11791,#11790,#7395,.T.);
#15701=EDGE_CURVE('',#11792,#11791,#7396,.T.);
#15702=EDGE_CURVE('',#11793,#11792,#6099,.T.);
#15703=EDGE_CURVE('',#11769,#11793,#7397,.T.);
#15704=EDGE_CURVE('',#11768,#11794,#6100,.T.);
#15705=EDGE_CURVE('',#11795,#11794,#6101,.T.);
#15706=EDGE_CURVE('',#11796,#11795,#7398,.T.);
#15707=EDGE_CURVE('',#11797,#11796,#6102,.T.);
#15708=EDGE_CURVE('',#11798,#11797,#7399,.T.);
#15709=EDGE_CURVE('',#11799,#11798,#6103,.T.);
#15710=EDGE_CURVE('',#11800,#11799,#7400,.T.);
#15711=EDGE_CURVE('',#11801,#11800,#6104,.T.);
#15712=EDGE_CURVE('',#11802,#11801,#7401,.T.);
#15713=EDGE_CURVE('',#11803,#11802,#6105,.T.);
#15714=EDGE_CURVE('',#11804,#11803,#7402,.T.);
#15715=EDGE_CURVE('',#11785,#11804,#6106,.T.);
#15716=EDGE_CURVE('',#11794,#11776,#7403,.T.);
#15717=EDGE_CURVE('',#11782,#11788,#7404,.T.);
#15718=EDGE_CURVE('',#11790,#11780,#7405,.F.);
#15719=EDGE_CURVE('',#11791,#11779,#7406,.F.);
#15720=EDGE_CURVE('',#11805,#11806,#7407,.F.);
#15721=EDGE_CURVE('',#11807,#11805,#7408,.F.);
#15722=EDGE_CURVE('',#11808,#11807,#7409,.F.);
#15723=EDGE_CURVE('',#11806,#11808,#7410,.F.);
#15724=EDGE_CURVE('',#11781,#11789,#7411,.T.);
#15725=EDGE_CURVE('',#11778,#11792,#7412,.T.);
#15726=EDGE_CURVE('',#11777,#11793,#7413,.T.);
#15727=EDGE_CURVE('',#11804,#11765,#7414,.T.);
#15728=EDGE_CURVE('',#11764,#11771,#7415,.F.);
#15729=EDGE_CURVE('',#11775,#11766,#7416,.F.);
#15730=EDGE_CURVE('',#11762,#11795,#7417,.T.);
#15731=EDGE_CURVE('',#11806,#11809,#7418,.F.);
#15732=EDGE_CURVE('',#11810,#11809,#7419,.T.);
#15733=EDGE_CURVE('',#11805,#11810,#7420,.F.);
#15734=EDGE_CURVE('',#11811,#11810,#7421,.T.);
#15735=EDGE_CURVE('',#11807,#11811,#7422,.F.);
#15736=EDGE_CURVE('',#11812,#11811,#7423,.T.);
#15737=EDGE_CURVE('',#11808,#11812,#7424,.F.);
#15738=EDGE_CURVE('',#11809,#11812,#7425,.T.);
#15739=EDGE_CURVE('',#11813,#11814,#7426,.T.);
#15740=EDGE_CURVE('',#11815,#11813,#6107,.T.);
#15741=EDGE_CURVE('',#11816,#11815,#7427,.T.);
#15742=EDGE_CURVE('',#11816,#11817,#6108,.T.);
#15743=EDGE_CURVE('',#11814,#11817,#7428,.T.);
#15744=EDGE_CURVE('',#11818,#11819,#7429,.T.);
#15745=EDGE_CURVE('',#11820,#11818,#7430,.T.);
#15746=EDGE_CURVE('',#11820,#11821,#6109,.T.);
#15747=EDGE_CURVE('',#11821,#11822,#7431,.T.);
#15748=EDGE_CURVE('',#11819,#11822,#6110,.T.);
#15749=EDGE_CURVE('',#11816,#11801,#7432,.T.);
#15750=EDGE_CURVE('',#11817,#11800,#7433,.T.);
#15751=EDGE_CURVE('',#11815,#11802,#7434,.T.);
#15752=EDGE_CURVE('',#11813,#11803,#7435,.T.);
#15753=EDGE_CURVE('',#11822,#11797,#7436,.T.);
#15754=EDGE_CURVE('',#11819,#11796,#7437,.T.);
#15755=EDGE_CURVE('',#11821,#11798,#7438,.T.);
#15756=EDGE_CURVE('',#11820,#11799,#7439,.T.);
#15757=EDGE_CURVE('',#11823,#11824,#7440,.T.);
#15758=EDGE_CURVE('',#11825,#11823,#6111,.T.);
#15759=EDGE_CURVE('',#11824,#11825,#7441,.F.);
#15760=EDGE_CURVE('',#11826,#11827,#7442,.T.);
#15761=EDGE_CURVE('',#11828,#11826,#7443,.T.);
#15762=EDGE_CURVE('',#11827,#11828,#6112,.T.);
#15763=EDGE_CURVE('',#11823,#11829,#6113,.T.);
#15764=EDGE_CURVE('',#11829,#11823,#7444,.T.);
#15765=EDGE_CURVE('',#11827,#11830,#7445,.F.);
#15766=EDGE_CURVE('',#11831,#11830,#7446,.T.);
#15767=EDGE_CURVE('',#11831,#11773,#7447,.T.);
#15768=EDGE_CURVE('',#11826,#11763,#7448,.F.);
#15769=EDGE_CURVE('',#11832,#11833,#7449,.T.);
#15770=EDGE_CURVE('',#11832,#11834,#7450,.T.);
#15771=EDGE_CURVE('',#11835,#11834,#7451,.F.);
#15772=EDGE_CURVE('',#11833,#11835,#7452,.T.);
#15773=EDGE_CURVE('',#11830,#11836,#6114,.T.);
#15774=EDGE_CURVE('',#11836,#11837,#6115,.T.);
#15775=EDGE_CURVE('',#11837,#11838,#7453,.F.);
#15776=EDGE_CURVE('',#11838,#11839,#7454,.F.);
#15777=EDGE_CURVE('',#11840,#11839,#6116,.T.);
#15778=EDGE_CURVE('',#11840,#11841,#7455,.F.);
#15779=EDGE_CURVE('',#11841,#11842,#7456,.F.);
#15780=EDGE_CURVE('',#11843,#11842,#7457,.T.);
#15781=EDGE_CURVE('',#11844,#11843,#6117,.T.);
#15782=EDGE_CURVE('',#11834,#11844,#7458,.T.);
#15783=EDGE_CURVE('',#11832,#11845,#6118,.T.);
#15784=EDGE_CURVE('',#11845,#11846,#6119,.T.);
#15785=EDGE_CURVE('',#11846,#11847,#7459,.T.);
#15786=EDGE_CURVE('',#11847,#11831,#7460,.T.);
#15787=EDGE_CURVE('',#11846,#11829,#7461,.F.);
#15788=EDGE_CURVE('',#11824,#11761,#7462,.T.);
#15789=EDGE_CURVE('',#11847,#11774,#7463,.F.);
#15790=EDGE_CURVE('',#11848,#11849,#6120,.T.);
#15791=EDGE_CURVE('',#11837,#11849,#7464,.T.);
#15792=EDGE_CURVE('',#11848,#11836,#7465,.T.);
#15793=EDGE_CURVE('',#11850,#11849,#7466,.T.);
#15794=EDGE_CURVE('',#11850,#11838,#7467,.F.);
#15795=EDGE_CURVE('',#11848,#11851,#6121,.T.);
#15796=EDGE_CURVE('',#11851,#11852,#7468,.T.);
#15797=EDGE_CURVE('',#11852,#11853,#6122,.T.);
#15798=EDGE_CURVE('',#11853,#11854,#7469,.T.);
#15799=EDGE_CURVE('',#11854,#11855,#6123,.T.);
#15800=EDGE_CURVE('',#11855,#11856,#7470,.T.);
#15801=EDGE_CURVE('',#11856,#11857,#6124,.T.);
#15802=EDGE_CURVE('',#11857,#11858,#7471,.T.);
#15803=EDGE_CURVE('',#11858,#11859,#6125,.T.);
#15804=EDGE_CURVE('',#11859,#11860,#7472,.T.);
#15805=EDGE_CURVE('',#11860,#11861,#6126,.T.);
#15806=EDGE_CURVE('',#11833,#11861,#6127,.T.);
#15807=EDGE_CURVE('',#11835,#11862,#7473,.T.);
#15808=EDGE_CURVE('',#11862,#11863,#6128,.T.);
#15809=EDGE_CURVE('',#11863,#11864,#7474,.T.);
#15810=EDGE_CURVE('',#11864,#11865,#7475,.T.);
#15811=EDGE_CURVE('',#11865,#11866,#7476,.T.);
#15812=EDGE_CURVE('',#11866,#11867,#6129,.T.);
#15813=EDGE_CURVE('',#11867,#11850,#7477,.T.);
#15814=EDGE_CURVE('',#11868,#11813,#7478,.T.);
#15815=EDGE_CURVE('',#11868,#11852,#7479,.T.);
#15816=EDGE_CURVE('',#11851,#11828,#7480,.T.);
#15817=EDGE_CURVE('',#11861,#11845,#7481,.T.);
#15818=EDGE_CURVE('',#11839,#11867,#7482,.T.);
#15819=EDGE_CURVE('',#11864,#11842,#7483,.F.);
#15820=EDGE_CURVE('',#11865,#11841,#7484,.F.);
#15821=EDGE_CURVE('',#11869,#11870,#7485,.F.);
#15822=EDGE_CURVE('',#11870,#11871,#7486,.F.);
#15823=EDGE_CURVE('',#11871,#11872,#7487,.F.);
#15824=EDGE_CURVE('',#11872,#11869,#7488,.F.);
#15825=EDGE_CURVE('',#11840,#11866,#7489,.T.);
#15826=EDGE_CURVE('',#11843,#11863,#7490,.T.);
#15827=EDGE_CURVE('',#11844,#11862,#7491,.T.);
#15828=EDGE_CURVE('',#11825,#11860,#7492,.T.);
#15829=EDGE_CURVE('',#11869,#11873,#7493,.F.);
#15830=EDGE_CURVE('',#11873,#11874,#7494,.T.);
#15831=EDGE_CURVE('',#11870,#11874,#7495,.F.);
#15832=EDGE_CURVE('',#11872,#11875,#7496,.F.);
#15833=EDGE_CURVE('',#11875,#11873,#7497,.T.);
#15834=EDGE_CURVE('',#11871,#11876,#7498,.F.);
#15835=EDGE_CURVE('',#11876,#11875,#7499,.T.);
#15836=EDGE_CURVE('',#11874,#11876,#7500,.T.);
#15837=EDGE_CURVE('',#11868,#11877,#7501,.T.);
#15838=EDGE_CURVE('',#11814,#11877,#7502,.T.);
#15839=EDGE_CURVE('',#11878,#11879,#7503,.T.);
#15840=EDGE_CURVE('',#11818,#11878,#7504,.T.);
#15841=EDGE_CURVE('',#11879,#11819,#7505,.T.);
#15842=EDGE_CURVE('',#11877,#11880,#7506,.T.);
#15843=EDGE_CURVE('',#11881,#11880,#6130,.T.);
#15844=EDGE_CURVE('',#11881,#11882,#7507,.T.);
#15845=EDGE_CURVE('',#11882,#11868,#6131,.T.);
#15846=EDGE_CURVE('',#11879,#11883,#6132,.T.);
#15847=EDGE_CURVE('',#11884,#11883,#7508,.T.);
#15848=EDGE_CURVE('',#11885,#11884,#6133,.T.);
#15849=EDGE_CURVE('',#11885,#11878,#7509,.T.);
#15850=EDGE_CURVE('',#11879,#11859,#7510,.T.);
#15851=EDGE_CURVE('',#11885,#11856,#7511,.T.);
#15852=EDGE_CURVE('',#11880,#11855,#7512,.T.);
#15853=EDGE_CURVE('',#11881,#11854,#7513,.T.);
#15854=EDGE_CURVE('',#11882,#11853,#7514,.T.);
#15855=EDGE_CURVE('',#11883,#11858,#7515,.T.);
#15856=EDGE_CURVE('',#11884,#11857,#7516,.T.);
#22607=ORIENTED_EDGE('',*,*,#15665,.T.);
#22608=ORIENTED_EDGE('',*,*,#15666,.T.);
#22609=ORIENTED_EDGE('',*,*,#15667,.T.);
#22610=ORIENTED_EDGE('',*,*,#15668,.T.);
#22611=ORIENTED_EDGE('',*,*,#15669,.T.);
#22612=ORIENTED_EDGE('',*,*,#15670,.T.);
#22613=ORIENTED_EDGE('',*,*,#15671,.T.);
#22614=ORIENTED_EDGE('',*,*,#15672,.T.);
#22615=ORIENTED_EDGE('',*,*,#15673,.T.);
#22616=ORIENTED_EDGE('',*,*,#15674,.T.);
#22617=ORIENTED_EDGE('',*,*,#15675,.T.);
#22618=ORIENTED_EDGE('',*,*,#15676,.F.);
#22619=ORIENTED_EDGE('',*,*,#15677,.F.);
#22620=ORIENTED_EDGE('',*,*,#15678,.F.);
#22621=ORIENTED_EDGE('',*,*,#15679,.F.);
#22622=ORIENTED_EDGE('',*,*,#15680,.F.);
#22623=ORIENTED_EDGE('',*,*,#15681,.F.);
#22624=ORIENTED_EDGE('',*,*,#15682,.F.);
#22625=ORIENTED_EDGE('',*,*,#15676,.T.);
#22626=ORIENTED_EDGE('',*,*,#15683,.T.);
#22627=ORIENTED_EDGE('',*,*,#15684,.T.);
#22628=ORIENTED_EDGE('',*,*,#15685,.T.);
#22629=ORIENTED_EDGE('',*,*,#15686,.F.);
#22630=ORIENTED_EDGE('',*,*,#15687,.F.);
#22631=ORIENTED_EDGE('',*,*,#15688,.T.);
#22632=ORIENTED_EDGE('',*,*,#15689,.F.);
#22633=ORIENTED_EDGE('',*,*,#15690,.F.);
#22634=ORIENTED_EDGE('',*,*,#15691,.F.);
#22635=ORIENTED_EDGE('',*,*,#15692,.F.);
#22636=ORIENTED_EDGE('',*,*,#15693,.T.);
#22637=ORIENTED_EDGE('',*,*,#15691,.T.);
#22638=ORIENTED_EDGE('',*,*,#15694,.T.);
#22639=ORIENTED_EDGE('',*,*,#15694,.F.);
#22640=ORIENTED_EDGE('',*,*,#15690,.T.);
#22641=ORIENTED_EDGE('',*,*,#15695,.F.);
#22642=ORIENTED_EDGE('',*,*,#15696,.T.);
#22643=ORIENTED_EDGE('',*,*,#15692,.T.);
#22644=ORIENTED_EDGE('',*,*,#15696,.F.);
#22645=ORIENTED_EDGE('',*,*,#15697,.F.);
#22646=ORIENTED_EDGE('',*,*,#15698,.F.);
#22647=ORIENTED_EDGE('',*,*,#15699,.F.);
#22648=ORIENTED_EDGE('',*,*,#15700,.F.);
#22649=ORIENTED_EDGE('',*,*,#15701,.F.);
#22650=ORIENTED_EDGE('',*,*,#15702,.F.);
#22651=ORIENTED_EDGE('',*,*,#15703,.F.);
#22652=ORIENTED_EDGE('',*,*,#15674,.F.);
#22653=ORIENTED_EDGE('',*,*,#15704,.T.);
#22654=ORIENTED_EDGE('',*,*,#15705,.F.);
#22655=ORIENTED_EDGE('',*,*,#15706,.F.);
#22656=ORIENTED_EDGE('',*,*,#15707,.F.);
#22657=ORIENTED_EDGE('',*,*,#15708,.F.);
#22658=ORIENTED_EDGE('',*,*,#15709,.F.);
#22659=ORIENTED_EDGE('',*,*,#15710,.F.);
#22660=ORIENTED_EDGE('',*,*,#15711,.F.);
#22661=ORIENTED_EDGE('',*,*,#15712,.F.);
#22662=ORIENTED_EDGE('',*,*,#15713,.F.);
#22663=ORIENTED_EDGE('',*,*,#15714,.F.);
#22664=ORIENTED_EDGE('',*,*,#15715,.F.);
#22665=ORIENTED_EDGE('',*,*,#15704,.F.);
#22666=ORIENTED_EDGE('',*,*,#15673,.F.);
#22667=ORIENTED_EDGE('',*,*,#15682,.T.);
#22668=ORIENTED_EDGE('',*,*,#15716,.F.);
#22669=ORIENTED_EDGE('',*,*,#15697,.T.);
#22670=ORIENTED_EDGE('',*,*,#15695,.T.);
#22671=ORIENTED_EDGE('',*,*,#15689,.T.);
#22672=ORIENTED_EDGE('',*,*,#15717,.T.);
#22673=ORIENTED_EDGE('',*,*,#15700,.T.);
#22674=ORIENTED_EDGE('',*,*,#15718,.T.);
#22675=ORIENTED_EDGE('',*,*,#15686,.T.);
#22676=ORIENTED_EDGE('',*,*,#15719,.F.);
#22677=ORIENTED_EDGE('',*,*,#15720,.F.);
#22678=ORIENTED_EDGE('',*,*,#15721,.F.);
#22679=ORIENTED_EDGE('',*,*,#15722,.F.);
#22680=ORIENTED_EDGE('',*,*,#15723,.F.);
#22681=ORIENTED_EDGE('',*,*,#15718,.F.);
#22682=ORIENTED_EDGE('',*,*,#15699,.T.);
#22683=ORIENTED_EDGE('',*,*,#15724,.F.);
#22684=ORIENTED_EDGE('',*,*,#15687,.T.);
#22685=ORIENTED_EDGE('',*,*,#15701,.T.);
#22686=ORIENTED_EDGE('',*,*,#15719,.T.);
#22687=ORIENTED_EDGE('',*,*,#15685,.F.);
#22688=ORIENTED_EDGE('',*,*,#15725,.T.);
#22689=ORIENTED_EDGE('',*,*,#15675,.F.);
#22690=ORIENTED_EDGE('',*,*,#15703,.T.);
#22691=ORIENTED_EDGE('',*,*,#15726,.F.);
#22692=ORIENTED_EDGE('',*,*,#15683,.F.);
#22693=ORIENTED_EDGE('',*,*,#15693,.F.);
#22694=ORIENTED_EDGE('',*,*,#15715,.T.);
#22695=ORIENTED_EDGE('',*,*,#15727,.T.);
#22696=ORIENTED_EDGE('',*,*,#15669,.F.);
#22697=ORIENTED_EDGE('',*,*,#15728,.T.);
#22698=ORIENTED_EDGE('',*,*,#15677,.T.);
#22699=ORIENTED_EDGE('',*,*,#15716,.T.);
#22700=ORIENTED_EDGE('',*,*,#15681,.T.);
#22701=ORIENTED_EDGE('',*,*,#15729,.T.);
#22702=ORIENTED_EDGE('',*,*,#15671,.F.);
#22703=ORIENTED_EDGE('',*,*,#15667,.F.);
#22704=ORIENTED_EDGE('',*,*,#15730,.T.);
#22705=ORIENTED_EDGE('',*,*,#15705,.T.);
#22706=ORIENTED_EDGE('',*,*,#15720,.T.);
#22707=ORIENTED_EDGE('',*,*,#15731,.T.);
#22708=ORIENTED_EDGE('',*,*,#15732,.F.);
#22709=ORIENTED_EDGE('',*,*,#15733,.F.);
#22710=ORIENTED_EDGE('',*,*,#15721,.T.);
#22711=ORIENTED_EDGE('',*,*,#15733,.T.);
#22712=ORIENTED_EDGE('',*,*,#15734,.F.);
#22713=ORIENTED_EDGE('',*,*,#15735,.F.);
#22714=ORIENTED_EDGE('',*,*,#15722,.T.);
#22715=ORIENTED_EDGE('',*,*,#15735,.T.);
#22716=ORIENTED_EDGE('',*,*,#15736,.F.);
#22717=ORIENTED_EDGE('',*,*,#15737,.F.);
#22718=ORIENTED_EDGE('',*,*,#15723,.T.);
#22719=ORIENTED_EDGE('',*,*,#15737,.T.);
#22720=ORIENTED_EDGE('',*,*,#15738,.F.);
#22721=ORIENTED_EDGE('',*,*,#15731,.F.);
#22722=ORIENTED_EDGE('',*,*,#15738,.T.);
#22723=ORIENTED_EDGE('',*,*,#15736,.T.);
#22724=ORIENTED_EDGE('',*,*,#15734,.T.);
#22725=ORIENTED_EDGE('',*,*,#15732,.T.);
#22726=ORIENTED_EDGE('',*,*,#15739,.F.);
#22727=ORIENTED_EDGE('',*,*,#15740,.F.);
#22728=ORIENTED_EDGE('',*,*,#15741,.F.);
#22729=ORIENTED_EDGE('',*,*,#15742,.T.);
#22730=ORIENTED_EDGE('',*,*,#15743,.F.);
#22731=ORIENTED_EDGE('',*,*,#15744,.F.);
#22732=ORIENTED_EDGE('',*,*,#15745,.F.);
#22733=ORIENTED_EDGE('',*,*,#15746,.T.);
#22734=ORIENTED_EDGE('',*,*,#15747,.T.);
#22735=ORIENTED_EDGE('',*,*,#15748,.F.);
#22736=ORIENTED_EDGE('',*,*,#15742,.F.);
#22737=ORIENTED_EDGE('',*,*,#15749,.T.);
#22738=ORIENTED_EDGE('',*,*,#15711,.T.);
#22739=ORIENTED_EDGE('',*,*,#15750,.F.);
#22740=ORIENTED_EDGE('',*,*,#15741,.T.);
#22741=ORIENTED_EDGE('',*,*,#15751,.T.);
#22742=ORIENTED_EDGE('',*,*,#15712,.T.);
#22743=ORIENTED_EDGE('',*,*,#15749,.F.);
#22744=ORIENTED_EDGE('',*,*,#15740,.T.);
#22745=ORIENTED_EDGE('',*,*,#15752,.T.);
#22746=ORIENTED_EDGE('',*,*,#15713,.T.);
#22747=ORIENTED_EDGE('',*,*,#15751,.F.);
#22748=ORIENTED_EDGE('',*,*,#15688,.F.);
#22749=ORIENTED_EDGE('',*,*,#15724,.T.);
#22750=ORIENTED_EDGE('',*,*,#15698,.T.);
#22751=ORIENTED_EDGE('',*,*,#15717,.F.);
#22752=ORIENTED_EDGE('',*,*,#15684,.F.);
#22753=ORIENTED_EDGE('',*,*,#15726,.T.);
#22754=ORIENTED_EDGE('',*,*,#15702,.T.);
#22755=ORIENTED_EDGE('',*,*,#15725,.F.);
#22756=ORIENTED_EDGE('',*,*,#15748,.T.);
#22757=ORIENTED_EDGE('',*,*,#15753,.T.);
#22758=ORIENTED_EDGE('',*,*,#15707,.T.);
#22759=ORIENTED_EDGE('',*,*,#15754,.F.);
#22760=ORIENTED_EDGE('',*,*,#15747,.F.);
#22761=ORIENTED_EDGE('',*,*,#15755,.T.);
#22762=ORIENTED_EDGE('',*,*,#15708,.T.);
#22763=ORIENTED_EDGE('',*,*,#15753,.F.);
#22764=ORIENTED_EDGE('',*,*,#15746,.F.);
#22765=ORIENTED_EDGE('',*,*,#15756,.T.);
#22766=ORIENTED_EDGE('',*,*,#15709,.T.);
#22767=ORIENTED_EDGE('',*,*,#15755,.F.);
#22768=ORIENTED_EDGE('',*,*,#15757,.F.);
#22769=ORIENTED_EDGE('',*,*,#15758,.F.);
#22770=ORIENTED_EDGE('',*,*,#15759,.F.);
#22771=ORIENTED_EDGE('',*,*,#15760,.F.);
#22772=ORIENTED_EDGE('',*,*,#15761,.F.);
#22773=ORIENTED_EDGE('',*,*,#15762,.F.);
#22774=ORIENTED_EDGE('',*,*,#15763,.F.);
#22775=ORIENTED_EDGE('',*,*,#15764,.F.);
#22776=ORIENTED_EDGE('',*,*,#15760,.T.);
#22777=ORIENTED_EDGE('',*,*,#15765,.T.);
#22778=ORIENTED_EDGE('',*,*,#15766,.F.);
#22779=ORIENTED_EDGE('',*,*,#15767,.T.);
#22780=ORIENTED_EDGE('',*,*,#15678,.T.);
#22781=ORIENTED_EDGE('',*,*,#15728,.F.);
#22782=ORIENTED_EDGE('',*,*,#15668,.F.);
#22783=ORIENTED_EDGE('',*,*,#15768,.F.);
#22784=ORIENTED_EDGE('',*,*,#15769,.F.);
#22785=ORIENTED_EDGE('',*,*,#15770,.T.);
#22786=ORIENTED_EDGE('',*,*,#15771,.F.);
#22787=ORIENTED_EDGE('',*,*,#15772,.F.);
#22788=ORIENTED_EDGE('',*,*,#15773,.T.);
#22789=ORIENTED_EDGE('',*,*,#15774,.T.);
#22790=ORIENTED_EDGE('',*,*,#15775,.T.);
#22791=ORIENTED_EDGE('',*,*,#15776,.T.);
#22792=ORIENTED_EDGE('',*,*,#15777,.F.);
#22793=ORIENTED_EDGE('',*,*,#15778,.T.);
#22794=ORIENTED_EDGE('',*,*,#15779,.T.);
#22795=ORIENTED_EDGE('',*,*,#15780,.F.);
#22796=ORIENTED_EDGE('',*,*,#15781,.F.);
#22797=ORIENTED_EDGE('',*,*,#15782,.F.);
#22798=ORIENTED_EDGE('',*,*,#15770,.F.);
#22799=ORIENTED_EDGE('',*,*,#15783,.T.);
#22800=ORIENTED_EDGE('',*,*,#15784,.T.);
#22801=ORIENTED_EDGE('',*,*,#15785,.T.);
#22802=ORIENTED_EDGE('',*,*,#15786,.T.);
#22803=ORIENTED_EDGE('',*,*,#15766,.T.);
#22804=ORIENTED_EDGE('',*,*,#15787,.T.);
#22805=ORIENTED_EDGE('',*,*,#15764,.T.);
#22806=ORIENTED_EDGE('',*,*,#15757,.T.);
#22807=ORIENTED_EDGE('',*,*,#15788,.T.);
#22808=ORIENTED_EDGE('',*,*,#15665,.F.);
#22809=ORIENTED_EDGE('',*,*,#15672,.F.);
#22810=ORIENTED_EDGE('',*,*,#15729,.F.);
#22811=ORIENTED_EDGE('',*,*,#15680,.T.);
#22812=ORIENTED_EDGE('',*,*,#15789,.F.);
#22813=ORIENTED_EDGE('',*,*,#15785,.F.);
#22814=ORIENTED_EDGE('',*,*,#15790,.T.);
#22815=ORIENTED_EDGE('',*,*,#15791,.F.);
#22816=ORIENTED_EDGE('',*,*,#15774,.F.);
#22817=ORIENTED_EDGE('',*,*,#15792,.F.);
#22818=ORIENTED_EDGE('',*,*,#15791,.T.);
#22819=ORIENTED_EDGE('',*,*,#15793,.F.);
#22820=ORIENTED_EDGE('',*,*,#15794,.T.);
#22821=ORIENTED_EDGE('',*,*,#15775,.F.);
#22822=ORIENTED_EDGE('',*,*,#15790,.F.);
#22823=ORIENTED_EDGE('',*,*,#15795,.T.);
#22824=ORIENTED_EDGE('',*,*,#15796,.T.);
#22825=ORIENTED_EDGE('',*,*,#15797,.T.);
#22826=ORIENTED_EDGE('',*,*,#15798,.T.);
#22827=ORIENTED_EDGE('',*,*,#15799,.T.);
#22828=ORIENTED_EDGE('',*,*,#15800,.T.);
#22829=ORIENTED_EDGE('',*,*,#15801,.T.);
#22830=ORIENTED_EDGE('',*,*,#15802,.T.);
#22831=ORIENTED_EDGE('',*,*,#15803,.T.);
#22832=ORIENTED_EDGE('',*,*,#15804,.T.);
#22833=ORIENTED_EDGE('',*,*,#15805,.T.);
#22834=ORIENTED_EDGE('',*,*,#15806,.F.);
#22835=ORIENTED_EDGE('',*,*,#15772,.T.);
#22836=ORIENTED_EDGE('',*,*,#15807,.T.);
#22837=ORIENTED_EDGE('',*,*,#15808,.T.);
#22838=ORIENTED_EDGE('',*,*,#15809,.T.);
#22839=ORIENTED_EDGE('',*,*,#15810,.T.);
#22840=ORIENTED_EDGE('',*,*,#15811,.T.);
#22841=ORIENTED_EDGE('',*,*,#15812,.T.);
#22842=ORIENTED_EDGE('',*,*,#15813,.T.);
#22843=ORIENTED_EDGE('',*,*,#15793,.T.);
#22844=ORIENTED_EDGE('',*,*,#15761,.T.);
#22845=ORIENTED_EDGE('',*,*,#15768,.T.);
#22846=ORIENTED_EDGE('',*,*,#15670,.F.);
#22847=ORIENTED_EDGE('',*,*,#15727,.F.);
#22848=ORIENTED_EDGE('',*,*,#15714,.T.);
#22849=ORIENTED_EDGE('',*,*,#15752,.F.);
#22850=ORIENTED_EDGE('',*,*,#15814,.F.);
#22851=ORIENTED_EDGE('',*,*,#15815,.T.);
#22852=ORIENTED_EDGE('',*,*,#15796,.F.);
#22853=ORIENTED_EDGE('',*,*,#15816,.T.);
#22854=ORIENTED_EDGE('',*,*,#15806,.T.);
#22855=ORIENTED_EDGE('',*,*,#15817,.T.);
#22856=ORIENTED_EDGE('',*,*,#15783,.F.);
#22857=ORIENTED_EDGE('',*,*,#15769,.T.);
#22858=ORIENTED_EDGE('',*,*,#15813,.F.);
#22859=ORIENTED_EDGE('',*,*,#15818,.F.);
#22860=ORIENTED_EDGE('',*,*,#15776,.F.);
#22861=ORIENTED_EDGE('',*,*,#15794,.F.);
#22862=ORIENTED_EDGE('',*,*,#15810,.F.);
#22863=ORIENTED_EDGE('',*,*,#15819,.T.);
#22864=ORIENTED_EDGE('',*,*,#15779,.F.);
#22865=ORIENTED_EDGE('',*,*,#15820,.F.);
#22866=ORIENTED_EDGE('',*,*,#15821,.T.);
#22867=ORIENTED_EDGE('',*,*,#15822,.T.);
#22868=ORIENTED_EDGE('',*,*,#15823,.T.);
#22869=ORIENTED_EDGE('',*,*,#15824,.T.);
#22870=ORIENTED_EDGE('',*,*,#15820,.T.);
#22871=ORIENTED_EDGE('',*,*,#15778,.F.);
#22872=ORIENTED_EDGE('',*,*,#15825,.T.);
#22873=ORIENTED_EDGE('',*,*,#15811,.F.);
#22874=ORIENTED_EDGE('',*,*,#15809,.F.);
#22875=ORIENTED_EDGE('',*,*,#15826,.F.);
#22876=ORIENTED_EDGE('',*,*,#15780,.T.);
#22877=ORIENTED_EDGE('',*,*,#15819,.F.);
#22878=ORIENTED_EDGE('',*,*,#15771,.T.);
#22879=ORIENTED_EDGE('',*,*,#15782,.T.);
#22880=ORIENTED_EDGE('',*,*,#15827,.T.);
#22881=ORIENTED_EDGE('',*,*,#15807,.F.);
#22882=ORIENTED_EDGE('',*,*,#15792,.T.);
#22883=ORIENTED_EDGE('',*,*,#15773,.F.);
#22884=ORIENTED_EDGE('',*,*,#15765,.F.);
#22885=ORIENTED_EDGE('',*,*,#15762,.T.);
#22886=ORIENTED_EDGE('',*,*,#15816,.F.);
#22887=ORIENTED_EDGE('',*,*,#15795,.F.);
#22888=ORIENTED_EDGE('',*,*,#15817,.F.);
#22889=ORIENTED_EDGE('',*,*,#15805,.F.);
#22890=ORIENTED_EDGE('',*,*,#15828,.F.);
#22891=ORIENTED_EDGE('',*,*,#15758,.T.);
#22892=ORIENTED_EDGE('',*,*,#15763,.T.);
#22893=ORIENTED_EDGE('',*,*,#15787,.F.);
#22894=ORIENTED_EDGE('',*,*,#15784,.F.);
#22895=ORIENTED_EDGE('',*,*,#15821,.F.);
#22896=ORIENTED_EDGE('',*,*,#15829,.T.);
#22897=ORIENTED_EDGE('',*,*,#15830,.T.);
#22898=ORIENTED_EDGE('',*,*,#15831,.F.);
#22899=ORIENTED_EDGE('',*,*,#15824,.F.);
#22900=ORIENTED_EDGE('',*,*,#15832,.T.);
#22901=ORIENTED_EDGE('',*,*,#15833,.T.);
#22902=ORIENTED_EDGE('',*,*,#15829,.F.);
#22903=ORIENTED_EDGE('',*,*,#15823,.F.);
#22904=ORIENTED_EDGE('',*,*,#15834,.T.);
#22905=ORIENTED_EDGE('',*,*,#15835,.T.);
#22906=ORIENTED_EDGE('',*,*,#15832,.F.);
#22907=ORIENTED_EDGE('',*,*,#15822,.F.);
#22908=ORIENTED_EDGE('',*,*,#15831,.T.);
#22909=ORIENTED_EDGE('',*,*,#15836,.T.);
#22910=ORIENTED_EDGE('',*,*,#15834,.F.);
#22911=ORIENTED_EDGE('',*,*,#15836,.F.);
#22912=ORIENTED_EDGE('',*,*,#15830,.F.);
#22913=ORIENTED_EDGE('',*,*,#15833,.F.);
#22914=ORIENTED_EDGE('',*,*,#15835,.F.);
#22915=ORIENTED_EDGE('',*,*,#15786,.F.);
#22916=ORIENTED_EDGE('',*,*,#15789,.T.);
#22917=ORIENTED_EDGE('',*,*,#15679,.T.);
#22918=ORIENTED_EDGE('',*,*,#15767,.F.);
#22919=ORIENTED_EDGE('',*,*,#15837,.F.);
#22920=ORIENTED_EDGE('',*,*,#15814,.T.);
#22921=ORIENTED_EDGE('',*,*,#15739,.T.);
#22922=ORIENTED_EDGE('',*,*,#15838,.T.);
#22923=ORIENTED_EDGE('',*,*,#15839,.F.);
#22924=ORIENTED_EDGE('',*,*,#15840,.F.);
#22925=ORIENTED_EDGE('',*,*,#15744,.T.);
#22926=ORIENTED_EDGE('',*,*,#15841,.F.);
#22927=ORIENTED_EDGE('',*,*,#15837,.T.);
#22928=ORIENTED_EDGE('',*,*,#15842,.T.);
#22929=ORIENTED_EDGE('',*,*,#15843,.F.);
#22930=ORIENTED_EDGE('',*,*,#15844,.T.);
#22931=ORIENTED_EDGE('',*,*,#15845,.T.);
#22932=ORIENTED_EDGE('',*,*,#15839,.T.);
#22933=ORIENTED_EDGE('',*,*,#15846,.T.);
#22934=ORIENTED_EDGE('',*,*,#15847,.F.);
#22935=ORIENTED_EDGE('',*,*,#15848,.F.);
#22936=ORIENTED_EDGE('',*,*,#15849,.T.);
#22937=ORIENTED_EDGE('',*,*,#15828,.T.);
#22938=ORIENTED_EDGE('',*,*,#15804,.F.);
#22939=ORIENTED_EDGE('',*,*,#15850,.F.);
#22940=ORIENTED_EDGE('',*,*,#15841,.T.);
#22941=ORIENTED_EDGE('',*,*,#15754,.T.);
#22942=ORIENTED_EDGE('',*,*,#15706,.T.);
#22943=ORIENTED_EDGE('',*,*,#15730,.F.);
#22944=ORIENTED_EDGE('',*,*,#15666,.F.);
#22945=ORIENTED_EDGE('',*,*,#15788,.F.);
#22946=ORIENTED_EDGE('',*,*,#15759,.T.);
#22947=ORIENTED_EDGE('',*,*,#15851,.T.);
#22948=ORIENTED_EDGE('',*,*,#15800,.F.);
#22949=ORIENTED_EDGE('',*,*,#15852,.F.);
#22950=ORIENTED_EDGE('',*,*,#15842,.F.);
#22951=ORIENTED_EDGE('',*,*,#15838,.F.);
#22952=ORIENTED_EDGE('',*,*,#15743,.T.);
#22953=ORIENTED_EDGE('',*,*,#15750,.T.);
#22954=ORIENTED_EDGE('',*,*,#15710,.T.);
#22955=ORIENTED_EDGE('',*,*,#15756,.F.);
#22956=ORIENTED_EDGE('',*,*,#15745,.T.);
#22957=ORIENTED_EDGE('',*,*,#15840,.T.);
#22958=ORIENTED_EDGE('',*,*,#15849,.F.);
#22959=ORIENTED_EDGE('',*,*,#15843,.T.);
#22960=ORIENTED_EDGE('',*,*,#15852,.T.);
#22961=ORIENTED_EDGE('',*,*,#15799,.F.);
#22962=ORIENTED_EDGE('',*,*,#15853,.F.);
#22963=ORIENTED_EDGE('',*,*,#15844,.F.);
#22964=ORIENTED_EDGE('',*,*,#15853,.T.);
#22965=ORIENTED_EDGE('',*,*,#15798,.F.);
#22966=ORIENTED_EDGE('',*,*,#15854,.F.);
#22967=ORIENTED_EDGE('',*,*,#15845,.F.);
#22968=ORIENTED_EDGE('',*,*,#15854,.T.);
#22969=ORIENTED_EDGE('',*,*,#15797,.F.);
#22970=ORIENTED_EDGE('',*,*,#15815,.F.);
#22971=ORIENTED_EDGE('',*,*,#15777,.T.);
#22972=ORIENTED_EDGE('',*,*,#15818,.T.);
#22973=ORIENTED_EDGE('',*,*,#15812,.F.);
#22974=ORIENTED_EDGE('',*,*,#15825,.F.);
#22975=ORIENTED_EDGE('',*,*,#15781,.T.);
#22976=ORIENTED_EDGE('',*,*,#15826,.T.);
#22977=ORIENTED_EDGE('',*,*,#15808,.F.);
#22978=ORIENTED_EDGE('',*,*,#15827,.F.);
#22979=ORIENTED_EDGE('',*,*,#15846,.F.);
#22980=ORIENTED_EDGE('',*,*,#15850,.T.);
#22981=ORIENTED_EDGE('',*,*,#15803,.F.);
#22982=ORIENTED_EDGE('',*,*,#15855,.F.);
#22983=ORIENTED_EDGE('',*,*,#15847,.T.);
#22984=ORIENTED_EDGE('',*,*,#15855,.T.);
#22985=ORIENTED_EDGE('',*,*,#15802,.F.);
#22986=ORIENTED_EDGE('',*,*,#15856,.F.);
#22987=ORIENTED_EDGE('',*,*,#15848,.T.);
#22988=ORIENTED_EDGE('',*,*,#15856,.T.);
#22989=ORIENTED_EDGE('',*,*,#15801,.F.);
#22990=ORIENTED_EDGE('',*,*,#15851,.F.);
#26586=PLANE('',#29434);
#26587=PLANE('',#29436);
#26588=PLANE('',#29438);
#26589=PLANE('',#29440);
#26590=PLANE('',#29441);
#26591=PLANE('',#29450);
#26592=PLANE('',#29451);
#26593=PLANE('',#29462);
#26594=PLANE('',#29463);
#26595=PLANE('',#29464);
#26596=PLANE('',#29465);
#26597=PLANE('',#29466);
#26598=PLANE('',#29469);
#26599=PLANE('',#29470);
#26600=PLANE('',#29471);
#26601=PLANE('',#29472);
#26602=PLANE('',#29473);
#26603=PLANE('',#29474);
#26604=PLANE('',#29477);
#26605=PLANE('',#29481);
#26606=PLANE('',#29486);
#26607=PLANE('',#29488);
#26608=PLANE('',#29490);
#26609=PLANE('',#29492);
#26610=PLANE('',#29494);
#26611=PLANE('',#29495);
#26612=PLANE('',#29496);
#26613=PLANE('',#29503);
#26614=PLANE('',#29506);
#26615=PLANE('',#29507);
#26616=PLANE('',#29517);
#26617=PLANE('',#29519);
#26618=PLANE('',#29520);
#26619=PLANE('',#29521);
#26620=PLANE('',#29522);
#26621=PLANE('',#29523);
#26622=PLANE('',#29526);
#26623=PLANE('',#29527);
#26624=PLANE('',#29528);
#26625=PLANE('',#29529);
#26626=PLANE('',#29530);
#26627=PLANE('',#29531);
#26628=PLANE('',#29532);
#26629=PLANE('',#29533);
#26630=PLANE('',#29534);
#26631=PLANE('',#29537);
#26632=PLANE('',#29540);
#26633=PLANE('',#29541);
#26634=PLANE('',#29543);
#26635=PLANE('',#29548);
#27555=ADVANCED_FACE('',(#3752),#26586,.T.);
#27556=ADVANCED_FACE('',(#3753),#26587,.F.);
#27557=ADVANCED_FACE('',(#3754),#26588,.F.);
#27558=ADVANCED_FACE('',(#3755),#26589,.F.);
#27559=ADVANCED_FACE('',(#3756),#26590,.F.);
#27560=ADVANCED_FACE('',(#3757),#2632,.T.);
#27561=ADVANCED_FACE('',(#3758),#26591,.F.);
#27562=ADVANCED_FACE('',(#3759),#26592,.T.);
#27563=ADVANCED_FACE('',(#3760),#2633,.T.);
#27564=ADVANCED_FACE('',(#3761),#26593,.F.);
#27565=ADVANCED_FACE('',(#3762,#216),#26594,.F.);
#27566=ADVANCED_FACE('',(#3763),#26595,.F.);
#27567=ADVANCED_FACE('',(#3764),#26596,.F.);
#27568=ADVANCED_FACE('',(#3765),#26597,.F.);
#27569=ADVANCED_FACE('',(#3766),#2634,.F.);
#27570=ADVANCED_FACE('',(#3767),#2635,.F.);
#27571=ADVANCED_FACE('',(#3768),#26598,.F.);
#27572=ADVANCED_FACE('',(#3769),#26599,.F.);
#27573=ADVANCED_FACE('',(#3770),#26600,.F.);
#27574=ADVANCED_FACE('',(#3771),#26601,.F.);
#27575=ADVANCED_FACE('',(#3772),#26602,.T.);
#27576=ADVANCED_FACE('',(#3773),#26603,.F.);
#27577=ADVANCED_FACE('',(#3774),#26604,.F.);
#27578=ADVANCED_FACE('',(#3775),#2636,.F.);
#27579=ADVANCED_FACE('',(#3776),#26605,.F.);
#27580=ADVANCED_FACE('',(#3777),#2637,.T.);
#27581=ADVANCED_FACE('',(#3778),#2638,.F.);
#27582=ADVANCED_FACE('',(#3779),#2639,.F.);
#27583=ADVANCED_FACE('',(#3780),#2640,.T.);
#27584=ADVANCED_FACE('',(#3781),#26606,.F.);
#27585=ADVANCED_FACE('',(#3782),#2641,.F.);
#27586=ADVANCED_FACE('',(#3783),#26607,.F.);
#27587=ADVANCED_FACE('',(#3784),#26608,.T.);
#27588=ADVANCED_FACE('',(#3785),#26609,.T.);
#27589=ADVANCED_FACE('',(#3786),#26610,.T.);
#27590=ADVANCED_FACE('',(#3787),#26611,.T.);
#27591=ADVANCED_FACE('',(#3788),#26612,.T.);
#27592=ADVANCED_FACE('',(#3789),#26613,.T.);
#27593=ADVANCED_FACE('',(#3790),#2642,.T.);
#27594=ADVANCED_FACE('',(#3791),#26614,.T.);
#27595=ADVANCED_FACE('',(#3792),#26615,.F.);
#27596=ADVANCED_FACE('',(#3793),#26616,.T.);
#27597=ADVANCED_FACE('',(#3794),#2643,.T.);
#27598=ADVANCED_FACE('',(#3795),#26617,.T.);
#27599=ADVANCED_FACE('',(#3796,#217),#26618,.T.);
#27600=ADVANCED_FACE('',(#3797),#26619,.T.);
#27601=ADVANCED_FACE('',(#3798),#26620,.T.);
#27602=ADVANCED_FACE('',(#3799),#26621,.T.);
#27603=ADVANCED_FACE('',(#3800),#2644,.F.);
#27604=ADVANCED_FACE('',(#3801),#2645,.F.);
#27605=ADVANCED_FACE('',(#3802),#26622,.T.);
#27606=ADVANCED_FACE('',(#3803),#26623,.T.);
#27607=ADVANCED_FACE('',(#3804),#26624,.T.);
#27608=ADVANCED_FACE('',(#3805),#26625,.T.);
#27609=ADVANCED_FACE('',(#3806),#26626,.F.);
#27610=ADVANCED_FACE('',(#3807),#26627,.T.);
#27611=ADVANCED_FACE('',(#3808),#26628,.T.);
#27612=ADVANCED_FACE('',(#3809),#26629,.T.);
#27613=ADVANCED_FACE('',(#3810),#26630,.T.);
#27614=ADVANCED_FACE('',(#3811),#26631,.T.);
#27615=ADVANCED_FACE('',(#3812),#26632,.T.);
#27616=ADVANCED_FACE('',(#3813),#26633,.T.);
#27617=ADVANCED_FACE('',(#3814),#2646,.F.);
#27618=ADVANCED_FACE('',(#3815),#26634,.T.);
#27619=ADVANCED_FACE('',(#3816),#2647,.T.);
#27620=ADVANCED_FACE('',(#3817),#2648,.F.);
#27621=ADVANCED_FACE('',(#3818),#2649,.F.);
#27622=ADVANCED_FACE('',(#3819),#2650,.T.);
#27623=ADVANCED_FACE('',(#3820),#26635,.T.);
#27624=ADVANCED_FACE('',(#3821),#2651,.F.);
#28086=CLOSED_SHELL('',(#27555,#27556,#27557,#27558,#27559,#27560,#27561,
#27562,#27563,#27564,#27565,#27566,#27567,#27568,#27569,#27570,#27571,#27572,
#27573,#27574,#27575,#27576,#27577,#27578,#27579,#27580,#27581,#27582,#27583,
#27584,#27585,#27586,#27587,#27588,#27589,#27590,#27591,#27592,#27593,#27594,
#27595,#27596,#27597,#27598,#27599,#27600,#27601,#27602,#27603,#27604,#27605,
#27606,#27607,#27608,#27609,#27610,#27611,#27612,#27613,#27614,#27615,#27616,
#27617,#27618,#27619,#27620,#27621,#27622,#27623,#27624));
#29433=AXIS2_PLACEMENT_3D('',#127452,#33749,#33750);
#29434=AXIS2_PLACEMENT_3D('',#127453,#33751,#33752);
#29435=AXIS2_PLACEMENT_3D('',#127459,#33755,#33756);
#29436=AXIS2_PLACEMENT_3D('',#127460,#33757,#33758);
#29437=AXIS2_PLACEMENT_3D('',#127465,#33760,#33761);
#29438=AXIS2_PLACEMENT_3D('',#127467,#33763,#33764);
#29439=AXIS2_PLACEMENT_3D('',#127469,#33765,#33766);
#29440=AXIS2_PLACEMENT_3D('',#127471,#33768,#33769);
#29441=AXIS2_PLACEMENT_3D('',#127480,#33774,#33775);
#29442=AXIS2_PLACEMENT_3D('',#127483,#33776,#33777);
#29443=AXIS2_PLACEMENT_3D('',#127491,#33781,#33782);
#29444=AXIS2_PLACEMENT_3D('',#127492,#33783,#33784);
#29445=AXIS2_PLACEMENT_3D('',#127496,#33786,#33787);
#29446=AXIS2_PLACEMENT_3D('',#127504,#33791,#33792);
#29447=AXIS2_PLACEMENT_3D('',#127509,#33795,#33796);
#29448=AXIS2_PLACEMENT_3D('',#127510,#33797,#33798);
#29449=AXIS2_PLACEMENT_3D('',#127513,#33799,#33800);
#29450=AXIS2_PLACEMENT_3D('',#127516,#33803,#33804);
#29451=AXIS2_PLACEMENT_3D('',#127520,#33807,#33808);
#29452=AXIS2_PLACEMENT_3D('',#127524,#33810,#33811);
#29453=AXIS2_PLACEMENT_3D('',#127532,#33815,#33816);
#29454=AXIS2_PLACEMENT_3D('',#127535,#33818,#33819);
#29455=AXIS2_PLACEMENT_3D('',#127537,#33820,#33821);
#29456=AXIS2_PLACEMENT_3D('',#127541,#33823,#33824);
#29457=AXIS2_PLACEMENT_3D('',#127545,#33826,#33827);
#29458=AXIS2_PLACEMENT_3D('',#127549,#33829,#33830);
#29459=AXIS2_PLACEMENT_3D('',#127553,#33832,#33833);
#29460=AXIS2_PLACEMENT_3D('',#127556,#33835,#33836);
#29461=AXIS2_PLACEMENT_3D('',#127557,#33837,#33838);
#29462=AXIS2_PLACEMENT_3D('',#127559,#33840,#33841);
#29463=AXIS2_PLACEMENT_3D('',#127561,#33843,#33844);
#29464=AXIS2_PLACEMENT_3D('',#127572,#33851,#33852);
#29465=AXIS2_PLACEMENT_3D('',#127574,#33854,#33855);
#29466=AXIS2_PLACEMENT_3D('',#127576,#33857,#33858);
#29467=AXIS2_PLACEMENT_3D('',#127578,#33860,#33861);
#29468=AXIS2_PLACEMENT_3D('',#127581,#33864,#33865);
#29469=AXIS2_PLACEMENT_3D('',#127584,#33868,#33869);
#29470=AXIS2_PLACEMENT_3D('',#127590,#33873,#33874);
#29471=AXIS2_PLACEMENT_3D('',#127594,#33877,#33878);
#29472=AXIS2_PLACEMENT_3D('',#127598,#33881,#33882);
#29473=AXIS2_PLACEMENT_3D('',#127600,#33884,#33885);
#29474=AXIS2_PLACEMENT_3D('',#127601,#33886,#33887);
#29475=AXIS2_PLACEMENT_3D('',#127606,#33889,#33890);
#29476=AXIS2_PLACEMENT_3D('',#127610,#33892,#33893);
#29477=AXIS2_PLACEMENT_3D('',#127612,#33895,#33896);
#29478=AXIS2_PLACEMENT_3D('',#127619,#33899,#33900);
#29479=AXIS2_PLACEMENT_3D('',#127622,#33902,#33903);
#29480=AXIS2_PLACEMENT_3D('',#127623,#33904,#33905);
#29481=AXIS2_PLACEMENT_3D('',#127626,#33908,#33909);
#29482=AXIS2_PLACEMENT_3D('',#127628,#33911,#33912);
#29483=AXIS2_PLACEMENT_3D('',#127630,#33914,#33915);
#29484=AXIS2_PLACEMENT_3D('',#127631,#33916,#33917);
#29485=AXIS2_PLACEMENT_3D('',#127632,#33918,#33919);
#29486=AXIS2_PLACEMENT_3D('',#127635,#33922,#33923);
#29487=AXIS2_PLACEMENT_3D('',#127637,#33925,#33926);
#29488=AXIS2_PLACEMENT_3D('',#127639,#33928,#33929);
#29489=AXIS2_PLACEMENT_3D('',#127644,#33931,#33932);
#29490=AXIS2_PLACEMENT_3D('',#127646,#33934,#33935);
#29491=AXIS2_PLACEMENT_3D('',#127652,#33938,#33939);
#29492=AXIS2_PLACEMENT_3D('',#127653,#33940,#33941);
#29493=AXIS2_PLACEMENT_3D('',#127655,#33942,#33943);
#29494=AXIS2_PLACEMENT_3D('',#127657,#33945,#33946);
#29495=AXIS2_PLACEMENT_3D('',#127664,#33951,#33952);
#29496=AXIS2_PLACEMENT_3D('',#127673,#33957,#33958);
#29497=AXIS2_PLACEMENT_3D('',#127675,#33959,#33960);
#29498=AXIS2_PLACEMENT_3D('',#127677,#33961,#33962);
#29499=AXIS2_PLACEMENT_3D('',#127683,#33965,#33966);
#29500=AXIS2_PLACEMENT_3D('',#127691,#33970,#33971);
#29501=AXIS2_PLACEMENT_3D('',#127694,#33973,#33974);
#29502=AXIS2_PLACEMENT_3D('',#127696,#33975,#33976);
#29503=AXIS2_PLACEMENT_3D('',#127700,#33979,#33980);
#29504=AXIS2_PLACEMENT_3D('',#127704,#33984,#33985);
#29505=AXIS2_PLACEMENT_3D('',#127707,#33986,#33987);
#29506=AXIS2_PLACEMENT_3D('',#127710,#33990,#33991);
#29507=AXIS2_PLACEMENT_3D('',#127714,#33994,#33995);
#29508=AXIS2_PLACEMENT_3D('',#127716,#33996,#33997);
#29509=AXIS2_PLACEMENT_3D('',#127720,#33999,#34000);
#29510=AXIS2_PLACEMENT_3D('',#127724,#34002,#34003);
#29511=AXIS2_PLACEMENT_3D('',#127728,#34005,#34006);
#29512=AXIS2_PLACEMENT_3D('',#127732,#34008,#34009);
#29513=AXIS2_PLACEMENT_3D('',#127736,#34011,#34012);
#29514=AXIS2_PLACEMENT_3D('',#127737,#34013,#34014);
#29515=AXIS2_PLACEMENT_3D('',#127741,#34016,#34017);
#29516=AXIS2_PLACEMENT_3D('',#127749,#34021,#34022);
#29517=AXIS2_PLACEMENT_3D('',#127751,#34024,#34025);
#29518=AXIS2_PLACEMENT_3D('',#127756,#34029,#34030);
#29519=AXIS2_PLACEMENT_3D('',#127758,#34032,#34033);
#29520=AXIS2_PLACEMENT_3D('',#127760,#34035,#34036);
#29521=AXIS2_PLACEMENT_3D('',#127771,#34043,#34044);
#29522=AXIS2_PLACEMENT_3D('',#127773,#34046,#34047);
#29523=AXIS2_PLACEMENT_3D('',#127775,#34049,#34050);
#29524=AXIS2_PLACEMENT_3D('',#127777,#34052,#34053);
#29525=AXIS2_PLACEMENT_3D('',#127778,#34054,#34055);
#29526=AXIS2_PLACEMENT_3D('',#127780,#34057,#34058);
#29527=AXIS2_PLACEMENT_3D('',#127786,#34062,#34063);
#29528=AXIS2_PLACEMENT_3D('',#127790,#34066,#34067);
#29529=AXIS2_PLACEMENT_3D('',#127794,#34070,#34071);
#29530=AXIS2_PLACEMENT_3D('',#127796,#34073,#34074);
#29531=AXIS2_PLACEMENT_3D('',#127797,#34075,#34076);
#29532=AXIS2_PLACEMENT_3D('',#127798,#34077,#34078);
#29533=AXIS2_PLACEMENT_3D('',#127802,#34081,#34082);
#29534=AXIS2_PLACEMENT_3D('',#127808,#34086,#34087);
#29535=AXIS2_PLACEMENT_3D('',#127812,#34089,#34090);
#29536=AXIS2_PLACEMENT_3D('',#127815,#34092,#34093);
#29537=AXIS2_PLACEMENT_3D('',#127816,#34094,#34095);
#29538=AXIS2_PLACEMENT_3D('',#127818,#34096,#34097);
#29539=AXIS2_PLACEMENT_3D('',#127822,#34099,#34100);
#29540=AXIS2_PLACEMENT_3D('',#127824,#34102,#34103);
#29541=AXIS2_PLACEMENT_3D('',#127826,#34105,#34106);
#29542=AXIS2_PLACEMENT_3D('',#127829,#34109,#34110);
#29543=AXIS2_PLACEMENT_3D('',#127831,#34112,#34113);
#29544=AXIS2_PLACEMENT_3D('',#127833,#34115,#34116);
#29545=AXIS2_PLACEMENT_3D('',#127834,#34117,#34118);
#29546=AXIS2_PLACEMENT_3D('',#127835,#34119,#34120);
#29547=AXIS2_PLACEMENT_3D('',#127836,#34121,#34122);
#29548=AXIS2_PLACEMENT_3D('',#127838,#34124,#34125);
#29549=AXIS2_PLACEMENT_3D('',#127840,#34127,#34128);
#33749=DIRECTION('axis',(0.,0.,1.));
#33750=DIRECTION('refdir',(1.,0.,0.));
#33751=DIRECTION('center_axis',(0.,0.,-1.));
#33752=DIRECTION('ref_axis',(-1.,0.,0.));
#33753=DIRECTION('',(0.0182661827191965,-0.999833159366536,0.));
#33754=DIRECTION('',(1.,0.,0.));
#33755=DIRECTION('center_axis',(0.,0.,1.));
#33756=DIRECTION('ref_axis',(0.966963946635808,-0.254913173269844,0.));
#33757=DIRECTION('center_axis',(0.,0.,-1.));
#33758=DIRECTION('ref_axis',(-1.,0.,0.));
#33759=DIRECTION('',(0.,1.,0.));
#33760=DIRECTION('center_axis',(0.,0.,1.));
#33761=DIRECTION('ref_axis',(-0.406016680407563,0.913865665856215,0.));
#33762=DIRECTION('',(1.,0.,0.));
#33763=DIRECTION('center_axis',(0.,0.,-1.));
#33764=DIRECTION('ref_axis',(-1.,0.,0.));
#33765=DIRECTION('center_axis',(0.,0.,1.));
#33766=DIRECTION('ref_axis',(0.966963946635808,-0.254913173269844,0.));
#33767=DIRECTION('',(0.0182661827191965,-0.999833159366536,0.));
#33768=DIRECTION('center_axis',(1.,0.,0.));
#33769=DIRECTION('ref_axis',(0.,1.,0.));
#33770=DIRECTION('',(0.,0.,1.));
#33771=DIRECTION('',(0.,1.,0.));
#33772=DIRECTION('',(0.,0.,1.));
#33773=DIRECTION('',(0.,1.,0.));
#33774=DIRECTION('center_axis',(0.,0.,1.));
#33775=DIRECTION('ref_axis',(1.,0.,0.));
#33776=DIRECTION('center_axis',(0.,0.,-1.));
#33777=DIRECTION('ref_axis',(-0.406016680407563,0.913865665856215,0.));
#33778=DIRECTION('',(0.,-1.,0.));
#33779=DIRECTION('',(1.,0.,0.));
#33780=DIRECTION('',(-0.0182661827191965,0.999833159366536,0.));
#33781=DIRECTION('center_axis',(0.,0.,-1.));
#33782=DIRECTION('ref_axis',(0.966963946635808,-0.254913173269844,0.));
#33783=DIRECTION('center_axis',(0.,0.,1.));
#33784=DIRECTION('ref_axis',(-0.866549484750265,-0.499091164497079,0.));
#33785=DIRECTION('',(1.,0.,0.));
#33786=DIRECTION('center_axis',(0.,0.,1.));
#33787=DIRECTION('ref_axis',(0.,-1.,0.));
#33788=DIRECTION('',(0.,1.,0.));
#33789=DIRECTION('',(1.,0.,0.));
#33790=DIRECTION('',(0.,-1.,0.));
#33791=DIRECTION('center_axis',(0.,0.,1.));
#33792=DIRECTION('ref_axis',(-1.,0.,0.));
#33793=DIRECTION('',(1.,0.,0.));
#33794=DIRECTION('',(0.,-1.,0.));
#33795=DIRECTION('center_axis',(0.,0.,1.));
#33796=DIRECTION('ref_axis',(0.866549484750267,-0.499091164497075,0.));
#33797=DIRECTION('center_axis',(0.,0.,-1.));
#33798=DIRECTION('ref_axis',(0.866549484750267,-0.499091164497075,0.));
#33799=DIRECTION('center_axis',(0.,0.,1.));
#33800=DIRECTION('ref_axis',(0.866549484750267,-0.499091164497075,0.));
#33801=DIRECTION('',(0.,0.,-1.));
#33802=DIRECTION('',(0.,0.,1.));
#33803=DIRECTION('center_axis',(-1.,0.,0.));
#33804=DIRECTION('ref_axis',(0.,-1.,0.));
#33805=DIRECTION('',(0.,0.,1.));
#33806=DIRECTION('',(0.,-1.,0.));
#33807=DIRECTION('center_axis',(0.,0.,1.));
#33808=DIRECTION('ref_axis',(1.,0.,0.));
#33809=DIRECTION('',(1.,0.,0.));
#33810=DIRECTION('center_axis',(0.,0.,1.));
#33811=DIRECTION('ref_axis',(-1.,0.,0.));
#33812=DIRECTION('',(0.,-1.,0.));
#33813=DIRECTION('',(1.,0.,0.));
#33814=DIRECTION('',(0.,1.,0.));
#33815=DIRECTION('center_axis',(0.,0.,1.));
#33816=DIRECTION('ref_axis',(0.,-1.,0.));
#33817=DIRECTION('',(1.,0.,0.));
#33818=DIRECTION('center_axis',(0.,0.,1.));
#33819=DIRECTION('ref_axis',(-0.866549484750265,-0.499091164497079,0.));
#33820=DIRECTION('center_axis',(0.,0.,1.));
#33821=DIRECTION('ref_axis',(0.966963946635808,-0.254913173269844,0.));
#33822=DIRECTION('',(-1.,0.,0.));
#33823=DIRECTION('center_axis',(0.,0.,-1.));
#33824=DIRECTION('ref_axis',(0.,-1.,0.));
#33825=DIRECTION('',(0.,-1.,0.));
#33826=DIRECTION('center_axis',(0.,0.,1.));
#33827=DIRECTION('ref_axis',(0.,1.,0.));
#33828=DIRECTION('',(-1.,0.,0.));
#33829=DIRECTION('center_axis',(0.,0.,1.));
#33830=DIRECTION('ref_axis',(1.,0.,0.));
#33831=DIRECTION('',(0.,1.,0.));
#33832=DIRECTION('center_axis',(0.,0.,-1.));
#33833=DIRECTION('ref_axis',(-1.,0.,0.));
#33834=DIRECTION('',(-1.,0.,0.));
#33835=DIRECTION('center_axis',(0.,0.,1.));
#33836=DIRECTION('ref_axis',(-0.406016680407563,0.913865665856215,0.));
#33837=DIRECTION('center_axis',(0.,0.,-1.));
#33838=DIRECTION('ref_axis',(-0.866549484750265,-0.499091164497079,0.));
#33839=DIRECTION('',(0.,0.,-1.));
#33840=DIRECTION('center_axis',(0.,-1.,0.));
#33841=DIRECTION('ref_axis',(1.,0.,0.));
#33842=DIRECTION('',(0.,0.,1.));
#33843=DIRECTION('center_axis',(0.,-1.,0.));
#33844=DIRECTION('ref_axis',(1.,0.,0.));
#33845=DIRECTION('',(0.,0.,1.));
#33846=DIRECTION('',(0.,0.,1.));
#33847=DIRECTION('',(1.,0.,0.));
#33848=DIRECTION('',(-1.08845394571094E-16,0.,1.));
#33849=DIRECTION('',(-1.,0.,0.));
#33850=DIRECTION('',(-1.08845394571094E-16,0.,-1.));
#33851=DIRECTION('center_axis',(-1.,0.,0.));
#33852=DIRECTION('ref_axis',(0.,-1.,0.));
#33853=DIRECTION('',(0.,0.,1.));
#33854=DIRECTION('center_axis',(1.,0.,0.));
#33855=DIRECTION('ref_axis',(0.,1.,0.));
#33856=DIRECTION('',(0.,0.,1.));
#33857=DIRECTION('center_axis',(0.,-1.,0.));
#33858=DIRECTION('ref_axis',(1.,0.,0.));
#33859=DIRECTION('',(0.,0.,1.));
#33860=DIRECTION('center_axis',(0.,0.,1.));
#33861=DIRECTION('ref_axis',(-0.406016680407563,0.913865665856215,0.));
#33862=DIRECTION('',(0.,0.,-1.));
#33863=DIRECTION('',(0.,0.,-1.));
#33864=DIRECTION('center_axis',(0.,0.,1.));
#33865=DIRECTION('ref_axis',(0.966963946635808,-0.254913173269844,0.));
#33866=DIRECTION('',(0.,0.,1.));
#33867=DIRECTION('',(0.,0.,1.));
#33868=DIRECTION('center_axis',(0.,0.,1.));
#33869=DIRECTION('ref_axis',(-1.,0.,0.));
#33870=DIRECTION('',(0.,-1.,0.));
#33871=DIRECTION('',(-1.,0.,0.));
#33872=DIRECTION('',(0.,-1.,0.));
#33873=DIRECTION('center_axis',(-1.,0.,-1.08845394571094E-16));
#33874=DIRECTION('ref_axis',(1.08845394571094E-16,0.,-1.));
#33875=DIRECTION('',(1.08845394571094E-16,0.,-1.));
#33876=DIRECTION('',(0.,-1.,0.));
#33877=DIRECTION('center_axis',(0.,0.,-1.));
#33878=DIRECTION('ref_axis',(1.,0.,0.));
#33879=DIRECTION('',(1.,0.,0.));
#33880=DIRECTION('',(0.,-1.,0.));
#33881=DIRECTION('center_axis',(1.,0.,-1.08845394571094E-16));
#33882=DIRECTION('ref_axis',(1.08845394571094E-16,0.,1.));
#33883=DIRECTION('',(1.08845394571094E-16,0.,1.));
#33884=DIRECTION('center_axis',(0.,1.,0.));
#33885=DIRECTION('ref_axis',(0.,0.,1.));
#33886=DIRECTION('center_axis',(0.,0.,1.));
#33887=DIRECTION('ref_axis',(1.,0.,0.));
#33888=DIRECTION('',(0.,1.,0.));
#33889=DIRECTION('center_axis',(0.,0.,1.));
#33890=DIRECTION('ref_axis',(-1.,0.,0.));
#33891=DIRECTION('',(0.,-1.,0.));
#33892=DIRECTION('center_axis',(0.,0.,1.));
#33893=DIRECTION('ref_axis',(1.,0.,0.));
#33894=DIRECTION('',(-1.,0.,0.));
#33895=DIRECTION('center_axis',(0.,0.,1.));
#33896=DIRECTION('ref_axis',(1.,0.,0.));
#33897=DIRECTION('',(0.,-1.,0.));
#33898=DIRECTION('',(-1.,0.,0.));
#33899=DIRECTION('center_axis',(0.,0.,1.));
#33900=DIRECTION('ref_axis',(0.,1.,0.));
#33901=DIRECTION('',(0.,-1.,0.));
#33902=DIRECTION('center_axis',(0.,0.,1.));
#33903=DIRECTION('ref_axis',(0.,-1.,0.));
#33904=DIRECTION('center_axis',(0.,0.,-1.));
#33905=DIRECTION('ref_axis',(1.,0.,0.));
#33906=DIRECTION('',(0.,0.,1.));
#33907=DIRECTION('',(0.,0.,1.));
#33908=DIRECTION('center_axis',(1.,0.,0.));
#33909=DIRECTION('ref_axis',(0.,1.,0.));
#33910=DIRECTION('',(0.,0.,1.));
#33911=DIRECTION('center_axis',(0.,0.,-1.));
#33912=DIRECTION('ref_axis',(-1.,0.,0.));
#33913=DIRECTION('',(0.,0.,1.));
#33914=DIRECTION('center_axis',(0.,0.,-1.));
#33915=DIRECTION('ref_axis',(-1.,0.,0.));
#33916=DIRECTION('center_axis',(0.,0.,-1.));
#33917=DIRECTION('ref_axis',(0.,-1.,0.));
#33918=DIRECTION('center_axis',(0.,0.,-1.));
#33919=DIRECTION('ref_axis',(0.,-1.,0.));
#33920=DIRECTION('',(0.,0.,1.));
#33921=DIRECTION('',(0.,0.,1.));
#33922=DIRECTION('center_axis',(-1.,0.,0.));
#33923=DIRECTION('ref_axis',(0.,-1.,0.));
#33924=DIRECTION('',(0.,0.,1.));
#33925=DIRECTION('center_axis',(0.,0.,-1.));
#33926=DIRECTION('ref_axis',(0.,1.,0.));
#33927=DIRECTION('',(0.,0.,1.));
#33928=DIRECTION('center_axis',(0.,0.,-1.));
#33929=DIRECTION('ref_axis',(-1.,0.,0.));
#33930=DIRECTION('',(0.0182661827191965,-0.999833159366536,0.));
#33931=DIRECTION('center_axis',(0.,0.,1.));
#33932=DIRECTION('ref_axis',(0.966963946635808,-0.254913173269844,0.));
#33933=DIRECTION('',(1.,0.,0.));
#33934=DIRECTION('center_axis',(0.,0.,-1.));
#33935=DIRECTION('ref_axis',(-1.,0.,0.));
#33936=DIRECTION('',(0.,1.,0.));
#33937=DIRECTION('',(1.,0.,0.));
#33938=DIRECTION('center_axis',(0.,0.,1.));
#33939=DIRECTION('ref_axis',(-0.406016680407563,0.913865665856215,0.));
#33940=DIRECTION('center_axis',(0.,0.,-1.));
#33941=DIRECTION('ref_axis',(-1.,0.,0.));
#33942=DIRECTION('center_axis',(0.,0.,1.));
#33943=DIRECTION('ref_axis',(0.966963946635808,-0.254913173269844,0.));
#33944=DIRECTION('',(0.0182661827191965,-0.999833159366536,0.));
#33945=DIRECTION('center_axis',(1.,0.,0.));
#33946=DIRECTION('ref_axis',(0.,1.,0.));
#33947=DIRECTION('',(0.,0.,1.));
#33948=DIRECTION('',(0.,-1.,0.));
#33949=DIRECTION('',(0.,0.,1.));
#33950=DIRECTION('',(0.,0.,-1.));
#33951=DIRECTION('center_axis',(-1.,0.,0.));
#33952=DIRECTION('ref_axis',(0.,1.,0.));
#33953=DIRECTION('',(0.,0.,-1.));
#33954=DIRECTION('',(0.,1.,0.));
#33955=DIRECTION('',(0.,0.,-1.));
#33956=DIRECTION('',(0.,1.,0.));
#33957=DIRECTION('center_axis',(0.,0.,1.));
#33958=DIRECTION('ref_axis',(1.,0.,0.));
#33959=DIRECTION('center_axis',(0.,0.,-1.));
#33960=DIRECTION('ref_axis',(-0.406016680407563,0.913865665856215,0.));
#33961=DIRECTION('center_axis',(0.,0.,1.));
#33962=DIRECTION('ref_axis',(0.866549484750267,-0.499091164497075,0.));
#33963=DIRECTION('',(0.,-1.,0.));
#33964=DIRECTION('',(1.,0.,0.));
#33965=DIRECTION('center_axis',(0.,0.,1.));
#33966=DIRECTION('ref_axis',(-1.,0.,0.));
#33967=DIRECTION('',(0.,-1.,0.));
#33968=DIRECTION('',(1.,0.,0.));
#33969=DIRECTION('',(0.,1.,0.));
#33970=DIRECTION('center_axis',(0.,0.,1.));
#33971=DIRECTION('ref_axis',(0.,-1.,0.));
#33972=DIRECTION('',(1.,0.,0.));
#33973=DIRECTION('center_axis',(0.,0.,1.));
#33974=DIRECTION('ref_axis',(-0.866549484750265,-0.499091164497079,0.));
#33975=DIRECTION('center_axis',(0.,0.,-1.));
#33976=DIRECTION('ref_axis',(0.966963946635808,-0.254913173269844,0.));
#33977=DIRECTION('',(-0.0182661827191965,0.999833159366536,0.));
#33978=DIRECTION('',(1.,0.,0.));
#33979=DIRECTION('center_axis',(-0.999833159366536,-0.0182661827191965,
0.));
#33980=DIRECTION('ref_axis',(0.0182661827191965,-0.999833159366536,0.));
#33981=DIRECTION('',(0.,0.,-1.));
#33982=DIRECTION('',(0.,0.,1.));
#33983=DIRECTION('',(0.,0.,-1.));
#33984=DIRECTION('center_axis',(0.,0.,-1.));
#33985=DIRECTION('ref_axis',(0.866549484750267,-0.499091164497075,0.));
#33986=DIRECTION('center_axis',(0.,0.,1.));
#33987=DIRECTION('ref_axis',(0.866549484750267,-0.499091164497075,0.));
#33988=DIRECTION('',(0.,0.,-1.));
#33989=DIRECTION('',(0.,0.,1.));
#33990=DIRECTION('center_axis',(1.,0.,0.));
#33991=DIRECTION('ref_axis',(0.,-1.,0.));
#33992=DIRECTION('',(0.,-1.,0.));
#33993=DIRECTION('',(0.,0.,-1.));
#33994=DIRECTION('center_axis',(0.,0.,1.));
#33995=DIRECTION('ref_axis',(1.,0.,0.));
#33996=DIRECTION('center_axis',(0.,0.,1.));
#33997=DIRECTION('ref_axis',(-0.406016680407563,0.913865665856215,0.));
#33998=DIRECTION('',(-1.,0.,0.));
#33999=DIRECTION('center_axis',(0.,0.,-1.));
#34000=DIRECTION('ref_axis',(-1.,0.,0.));
#34001=DIRECTION('',(0.,1.,0.));
#34002=DIRECTION('center_axis',(0.,0.,1.));
#34003=DIRECTION('ref_axis',(1.,0.,0.));
#34004=DIRECTION('',(-1.,0.,0.));
#34005=DIRECTION('center_axis',(0.,0.,1.));
#34006=DIRECTION('ref_axis',(0.,1.,0.));
#34007=DIRECTION('',(0.,-1.,0.));
#34008=DIRECTION('center_axis',(0.,0.,-1.));
#34009=DIRECTION('ref_axis',(0.,-1.,0.));
#34010=DIRECTION('',(-1.,0.,0.));
#34011=DIRECTION('center_axis',(0.,0.,1.));
#34012=DIRECTION('ref_axis',(0.966963946635808,-0.254913173269844,0.));
#34013=DIRECTION('center_axis',(0.,0.,1.));
#34014=DIRECTION('ref_axis',(-0.866549484750265,-0.499091164497079,0.));
#34015=DIRECTION('',(1.,0.,0.));
#34016=DIRECTION('center_axis',(0.,0.,1.));
#34017=DIRECTION('ref_axis',(0.,-1.,0.));
#34018=DIRECTION('',(0.,1.,0.));
#34019=DIRECTION('',(1.,0.,0.));
#34020=DIRECTION('',(0.,-1.,0.));
#34021=DIRECTION('center_axis',(0.,0.,1.));
#34022=DIRECTION('ref_axis',(-1.,0.,0.));
#34023=DIRECTION('',(1.,0.,0.));
#34024=DIRECTION('center_axis',(0.,-1.,0.));
#34025=DIRECTION('ref_axis',(-1.,0.,0.));
#34026=DIRECTION('',(0.,0.,1.));
#34027=DIRECTION('',(0.,0.,-1.));
#34028=DIRECTION('',(0.,0.,1.));
#34029=DIRECTION('center_axis',(0.,0.,-1.));
#34030=DIRECTION('ref_axis',(-0.866549484750265,-0.499091164497079,0.));
#34031=DIRECTION('',(0.,0.,1.));
#34032=DIRECTION('center_axis',(0.,1.,0.));
#34033=DIRECTION('ref_axis',(1.,0.,0.));
#34034=DIRECTION('',(0.,0.,-1.));
#34035=DIRECTION('center_axis',(0.,1.,0.));
#34036=DIRECTION('ref_axis',(1.,0.,0.));
#34037=DIRECTION('',(0.,0.,-1.));
#34038=DIRECTION('',(0.,0.,-1.));
#34039=DIRECTION('',(1.,0.,0.));
#34040=DIRECTION('',(-1.08845394571094E-16,0.,1.));
#34041=DIRECTION('',(-1.,0.,0.));
#34042=DIRECTION('',(-1.08845394571094E-16,0.,-1.));
#34043=DIRECTION('center_axis',(1.,0.,0.));
#34044=DIRECTION('ref_axis',(0.,-1.,0.));
#34045=DIRECTION('',(0.,0.,-1.));
#34046=DIRECTION('center_axis',(-1.,0.,0.));
#34047=DIRECTION('ref_axis',(0.,1.,0.));
#34048=DIRECTION('',(0.,0.,-1.));
#34049=DIRECTION('center_axis',(0.,1.,0.));
#34050=DIRECTION('ref_axis',(1.,0.,0.));
#34051=DIRECTION('',(0.,0.,-1.));
#34052=DIRECTION('center_axis',(0.,0.,1.));
#34053=DIRECTION('ref_axis',(-0.406016680407563,0.913865665856215,0.));
#34054=DIRECTION('center_axis',(0.,0.,1.));
#34055=DIRECTION('ref_axis',(0.966963946635808,-0.254913173269844,0.));
#34056=DIRECTION('',(0.,0.,-1.));
#34057=DIRECTION('center_axis',(0.,0.,1.));
#34058=DIRECTION('ref_axis',(-1.,0.,0.));
#34059=DIRECTION('',(0.,-1.,0.));
#34060=DIRECTION('',(-1.,0.,0.));
#34061=DIRECTION('',(0.,-1.,0.));
#34062=DIRECTION('center_axis',(1.,0.,-1.08845394571094E-16));
#34063=DIRECTION('ref_axis',(1.08845394571094E-16,0.,1.));
#34064=DIRECTION('',(0.,-1.,0.));
#34065=DIRECTION('',(1.08845394571094E-16,0.,1.));
#34066=DIRECTION('center_axis',(0.,0.,-1.));
#34067=DIRECTION('ref_axis',(1.,0.,0.));
#34068=DIRECTION('',(0.,-1.,0.));
#34069=DIRECTION('',(1.,0.,0.));
#34070=DIRECTION('center_axis',(-1.,0.,-1.08845394571094E-16));
#34071=DIRECTION('ref_axis',(1.08845394571094E-16,0.,-1.));
#34072=DIRECTION('',(1.08845394571094E-16,0.,-1.));
#34073=DIRECTION('center_axis',(0.,-1.,0.));
#34074=DIRECTION('ref_axis',(0.,0.,-1.));
#34075=DIRECTION('center_axis',(0.,1.,0.));
#34076=DIRECTION('ref_axis',(-1.,0.,0.));
#34077=DIRECTION('center_axis',(-1.,0.,0.));
#34078=DIRECTION('ref_axis',(0.,-1.,0.));
#34079=DIRECTION('',(0.,1.,0.));
#34080=DIRECTION('',(0.,0.,-1.));
#34081=DIRECTION('center_axis',(1.,0.,0.));
#34082=DIRECTION('ref_axis',(0.,1.,0.));
#34083=DIRECTION('',(0.,-1.,0.));
#34084=DIRECTION('',(0.,0.,-1.));
#34085=DIRECTION('',(0.,0.,1.));
#34086=DIRECTION('center_axis',(0.,0.,1.));
#34087=DIRECTION('ref_axis',(1.,0.,0.));
#34088=DIRECTION('',(-1.,0.,0.));
#34089=DIRECTION('center_axis',(0.,0.,1.));
#34090=DIRECTION('ref_axis',(1.,0.,0.));
#34091=DIRECTION('',(0.,-1.,0.));
#34092=DIRECTION('center_axis',(0.,0.,1.));
#34093=DIRECTION('ref_axis',(-1.,0.,0.));
#34094=DIRECTION('center_axis',(0.,0.,1.));
#34095=DIRECTION('ref_axis',(1.,0.,0.));
#34096=DIRECTION('center_axis',(0.,0.,1.));
#34097=DIRECTION('ref_axis',(0.,-1.,0.));
#34098=DIRECTION('',(0.,-1.,0.));
#34099=DIRECTION('center_axis',(0.,0.,1.));
#34100=DIRECTION('ref_axis',(0.,1.,0.));
#34101=DIRECTION('',(-1.,0.,0.));
#34102=DIRECTION('center_axis',(0.,-1.,0.));
#34103=DIRECTION('ref_axis',(-1.,0.,0.));
#34104=DIRECTION('',(0.,0.,-1.));
#34105=DIRECTION('center_axis',(0.,-1.,0.));
#34106=DIRECTION('ref_axis',(-1.,0.,0.));
#34107=DIRECTION('',(0.,0.,-1.));
#34108=DIRECTION('',(0.,0.,-1.));
#34109=DIRECTION('center_axis',(0.,0.,-1.));
#34110=DIRECTION('ref_axis',(1.,0.,0.));
#34111=DIRECTION('',(0.,0.,-1.));
#34112=DIRECTION('center_axis',(-1.,0.,0.));
#34113=DIRECTION('ref_axis',(0.,1.,0.));
#34114=DIRECTION('',(0.,0.,-1.));
#34115=DIRECTION('center_axis',(0.,0.,-1.));
#34116=DIRECTION('ref_axis',(-1.,0.,0.));
#34117=DIRECTION('center_axis',(0.,0.,-1.));
#34118=DIRECTION('ref_axis',(-1.,0.,0.));
#34119=DIRECTION('center_axis',(0.,0.,-1.));
#34120=DIRECTION('ref_axis',(0.,-1.,0.));
#34121=DIRECTION('center_axis',(0.,0.,-1.));
#34122=DIRECTION('ref_axis',(0.,-1.,0.));
#34123=DIRECTION('',(0.,0.,-1.));
#34124=DIRECTION('center_axis',(1.,0.,0.));
#34125=DIRECTION('ref_axis',(0.,-1.,0.));
#34126=DIRECTION('',(0.,0.,-1.));
#34127=DIRECTION('center_axis',(0.,0.,-1.));
#34128=DIRECTION('ref_axis',(0.,1.,0.));
#127452=CARTESIAN_POINT('',(0.,0.,0.));
#127453=CARTESIAN_POINT('Origin',(0.,17.2745,396.));
#127454=CARTESIAN_POINT('',(-6.81246236636335,15.2682931400241,396.));
#127455=CARTESIAN_POINT('',(-6.80496662630522,14.858,396.));
#127456=CARTESIAN_POINT('',(-6.87343118006261,18.6055334688258,396.));
#127457=CARTESIAN_POINT('',(-6.89783581472438,14.858,396.));
#127458=CARTESIAN_POINT('',(-2.477,14.858,396.));
#127459=CARTESIAN_POINT('Origin',(-10.752,15.874,396.));
#127460=CARTESIAN_POINT('Origin',(0.,17.2745,396.));
#127461=CARTESIAN_POINT('',(6.9,14.858,396.));
#127462=CARTESIAN_POINT('',(6.9000000000081,16.898174578473,396.));
#127463=CARTESIAN_POINT('',(6.9,16.06625,396.));
#127464=CARTESIAN_POINT('',(6.89783581472438,14.858,396.));
#127465=CARTESIAN_POINT('Origin',(10.752,15.874,396.));
#127466=CARTESIAN_POINT('',(-2.477,14.858,396.));
#127467=CARTESIAN_POINT('Origin',(0.,17.2745,396.));
#127468=CARTESIAN_POINT('',(-6.83721545938402,16.6231992843132,396.));
#127469=CARTESIAN_POINT('Origin',(-10.752,15.874,396.));
#127470=CARTESIAN_POINT('',(-6.87343118006261,18.6055334688258,396.));
#127471=CARTESIAN_POINT('Origin',(-8.847,15.049,400.));
#127472=CARTESIAN_POINT('',(-8.847,19.4868506020415,400.));
#127473=CARTESIAN_POINT('',(-8.847,19.4868506020415,422.));
#127474=CARTESIAN_POINT('',(-8.847,19.4868506020415,416.));
#127475=CARTESIAN_POINT('',(-8.847,22.145,422.));
#127476=CARTESIAN_POINT('',(-8.847,17.27175,422.));
#127477=CARTESIAN_POINT('',(-8.847,22.145,400.));
#127478=CARTESIAN_POINT('',(-8.847,22.145,400.));
#127479=CARTESIAN_POINT('',(-8.847,17.27175,400.));
#127480=CARTESIAN_POINT('Origin',(0.,19.4945,400.));
#127481=CARTESIAN_POINT('',(6.9000000000081,16.898174578473,400.));
#127482=CARTESIAN_POINT('',(8.751846859637,19.321640494912,400.));
#127483=CARTESIAN_POINT('Origin',(10.752,15.874,400.));
#127484=CARTESIAN_POINT('',(6.9,20.058,400.));
#127485=CARTESIAN_POINT('',(6.9,17.17625,400.));
#127486=CARTESIAN_POINT('',(-6.89996662630522,20.058,400.));
#127487=CARTESIAN_POINT('',(3.55,20.058,400.));
#127488=CARTESIAN_POINT('',(-6.83721545938402,16.6231992843132,400.));
#127489=CARTESIAN_POINT('',(-6.89370326010986,19.7151631135172,400.));
#127490=CARTESIAN_POINT('',(-8.751846859637,19.321640494912,400.));
#127491=CARTESIAN_POINT('Origin',(-10.752,15.874,400.));
#127492=CARTESIAN_POINT('Origin',(-8.656,19.4868506020415,400.));
#127493=CARTESIAN_POINT('',(-7.291,22.145,400.));
#127494=CARTESIAN_POINT('',(-4.528,22.145,400.));
#127495=CARTESIAN_POINT('',(-6.7,22.736,400.));
#127496=CARTESIAN_POINT('Origin',(-7.291,22.736,400.));
#127497=CARTESIAN_POINT('',(-6.7,23.731,400.));
#127498=CARTESIAN_POINT('',(-6.7,21.11525,400.));
#127499=CARTESIAN_POINT('',(6.7,23.731,400.));
#127500=CARTESIAN_POINT('',(-3.4545,23.731,400.));
#127501=CARTESIAN_POINT('',(6.7,22.736,400.));
#127502=CARTESIAN_POINT('',(6.7,21.71725,400.));
#127503=CARTESIAN_POINT('',(7.291,22.145,400.));
#127504=CARTESIAN_POINT('Origin',(7.291,22.736,400.));
#127505=CARTESIAN_POINT('',(8.847,22.145,400.));
#127506=CARTESIAN_POINT('',(3.6455,22.145,400.));
#127507=CARTESIAN_POINT('',(8.847,19.4868506020415,400.));
#127508=CARTESIAN_POINT('',(8.847,20.92425,400.));
#127509=CARTESIAN_POINT('Origin',(8.656,19.4868506020415,400.));
#127510=CARTESIAN_POINT('Origin',(8.656,19.4868506020415,422.));
#127511=CARTESIAN_POINT('',(8.751846859637,19.321640494912,422.));
#127512=CARTESIAN_POINT('',(8.847,19.4868506020415,422.));
#127513=CARTESIAN_POINT('Origin',(8.656,19.4868506020415,422.));
#127514=CARTESIAN_POINT('',(8.751846859637,19.321640494912,416.));
#127515=CARTESIAN_POINT('',(8.847,19.4868506020415,416.));
#127516=CARTESIAN_POINT('Origin',(8.847,22.354,400.));
#127517=CARTESIAN_POINT('',(8.847,22.145,422.));
#127518=CARTESIAN_POINT('',(8.847,22.145,400.));
#127519=CARTESIAN_POINT('',(8.847,20.92425,422.));
#127520=CARTESIAN_POINT('Origin',(0.,19.4945,422.));
#127521=CARTESIAN_POINT('',(7.291,22.145,422.));
#127522=CARTESIAN_POINT('',(3.6455,22.145,422.));
#127523=CARTESIAN_POINT('',(6.7,22.736,422.));
#127524=CARTESIAN_POINT('Origin',(7.291,22.736,422.));
#127525=CARTESIAN_POINT('',(6.7,23.731,422.));
#127526=CARTESIAN_POINT('',(6.7,21.71725,422.));
#127527=CARTESIAN_POINT('',(-6.7,23.731,422.));
#127528=CARTESIAN_POINT('',(-3.4545,23.731,422.));
#127529=CARTESIAN_POINT('',(-6.7,22.736,422.));
#127530=CARTESIAN_POINT('',(-6.7,21.11525,422.));
#127531=CARTESIAN_POINT('',(-7.291,22.145,422.));
#127532=CARTESIAN_POINT('Origin',(-7.291,22.736,422.));
#127533=CARTESIAN_POINT('',(-4.528,22.145,422.));
#127534=CARTESIAN_POINT('',(-8.751846859637,19.321640494912,422.));
#127535=CARTESIAN_POINT('Origin',(-8.656,19.4868506020415,422.));
#127536=CARTESIAN_POINT('',(-6.89783581472438,14.858,422.));
#127537=CARTESIAN_POINT('Origin',(-10.752,15.874,422.));
#127538=CARTESIAN_POINT('',(-4.954,14.858,422.));
#127539=CARTESIAN_POINT('',(-6.898,14.858,422.));
#127540=CARTESIAN_POINT('',(-4.763,15.049,422.));
#127541=CARTESIAN_POINT('Origin',(-4.954,15.049,422.));
#127542=CARTESIAN_POINT('',(-4.763,19.748,422.));
#127543=CARTESIAN_POINT('',(-4.763,19.748,422.));
#127544=CARTESIAN_POINT('',(-4.572,19.939,422.));
#127545=CARTESIAN_POINT('Origin',(-4.572,19.748,422.));
#127546=CARTESIAN_POINT('',(4.572,19.939,422.));
#127547=CARTESIAN_POINT('',(-4.572,19.939,422.));
#127548=CARTESIAN_POINT('',(4.763,19.748,422.));
#127549=CARTESIAN_POINT('Origin',(4.572,19.748,422.));
#127550=CARTESIAN_POINT('',(4.763,15.049,422.));
#127551=CARTESIAN_POINT('',(4.763,19.748,422.));
#127552=CARTESIAN_POINT('',(4.954,14.858,422.));
#127553=CARTESIAN_POINT('Origin',(4.954,15.049,422.));
#127554=CARTESIAN_POINT('',(6.89783581472438,14.858,422.));
#127555=CARTESIAN_POINT('',(4.954,14.858,422.));
#127556=CARTESIAN_POINT('Origin',(10.752,15.874,422.));
#127557=CARTESIAN_POINT('Origin',(-8.656,19.4868506020415,422.));
#127558=CARTESIAN_POINT('',(-8.751846859637,19.321640494912,422.));
#127559=CARTESIAN_POINT('Origin',(7.291,22.145,400.));
#127560=CARTESIAN_POINT('',(7.291,22.145,400.));
#127561=CARTESIAN_POINT('Origin',(-6.909,23.731,400.));
#127562=CARTESIAN_POINT('',(6.7,23.731,400.));
#127563=CARTESIAN_POINT('',(-6.7,23.731,400.));
#127564=CARTESIAN_POINT('',(6.109,23.731,400.8));
#127565=CARTESIAN_POINT('',(-6.109,23.731,400.8));
#127566=CARTESIAN_POINT('',(-0.399999999999999,23.731,400.8));
#127567=CARTESIAN_POINT('',(6.109,23.731,421.2));
#127568=CARTESIAN_POINT('',(6.109,23.731,410.6));
#127569=CARTESIAN_POINT('',(-6.109,23.731,421.2));
#127570=CARTESIAN_POINT('',(-6.509,23.731,421.2));
#127571=CARTESIAN_POINT('',(-6.109,23.731,400.4));
#127572=CARTESIAN_POINT('Origin',(6.7,23.94,400.));
#127573=CARTESIAN_POINT('',(6.7,22.736,400.));
#127574=CARTESIAN_POINT('Origin',(-6.7,22.736,400.));
#127575=CARTESIAN_POINT('',(-6.7,22.736,400.));
#127576=CARTESIAN_POINT('Origin',(-9.056,22.145,400.));
#127577=CARTESIAN_POINT('',(-7.291,22.145,400.));
#127578=CARTESIAN_POINT('Origin',(10.752,15.874,422.));
#127579=CARTESIAN_POINT('',(6.89783581472438,14.858,422.));
#127580=CARTESIAN_POINT('',(6.9,16.89817457841,422.));
#127581=CARTESIAN_POINT('Origin',(-10.752,15.874,422.));
#127582=CARTESIAN_POINT('',(-6.83721545938402,16.6231992843132,422.));
#127583=CARTESIAN_POINT('',(-6.89783581472438,14.858,422.));
#127584=CARTESIAN_POINT('Origin',(6.109,24.131,400.8));
#127585=CARTESIAN_POINT('',(-6.109,23.931,400.8));
#127586=CARTESIAN_POINT('',(-6.109,24.131,400.8));
#127587=CARTESIAN_POINT('',(6.109,23.931,400.8));
#127588=CARTESIAN_POINT('',(-6.109,23.931,400.8));
#127589=CARTESIAN_POINT('',(6.109,24.131,400.8));
#127590=CARTESIAN_POINT('Origin',(6.109,24.131,421.2));
#127591=CARTESIAN_POINT('',(6.109,23.931,421.2));
#127592=CARTESIAN_POINT('',(6.109,23.931,400.8));
#127593=CARTESIAN_POINT('',(6.109,24.131,421.2));
#127594=CARTESIAN_POINT('Origin',(-6.109,24.131,421.2));
#127595=CARTESIAN_POINT('',(-6.109,23.931,421.2));
#127596=CARTESIAN_POINT('',(6.109,23.931,421.2));
#127597=CARTESIAN_POINT('',(-6.109,24.131,421.2));
#127598=CARTESIAN_POINT('Origin',(-6.109,24.131,400.8));
#127599=CARTESIAN_POINT('',(-6.109,23.931,421.2));
#127600=CARTESIAN_POINT('Origin',(1.11022302462516E-15,23.931,411.));
#127601=CARTESIAN_POINT('Origin',(0.,19.4945,400.));
#127602=CARTESIAN_POINT('',(4.954,14.858,400.));
#127603=CARTESIAN_POINT('',(4.954,19.939,400.));
#127604=CARTESIAN_POINT('',(4.954,18.67625,400.));
#127605=CARTESIAN_POINT('',(4.763,15.049,400.));
#127606=CARTESIAN_POINT('Origin',(4.954,15.049,400.));
#127607=CARTESIAN_POINT('',(4.763,19.748,400.));
#127608=CARTESIAN_POINT('',(4.763,19.748,400.));
#127609=CARTESIAN_POINT('',(4.572,19.939,400.));
#127610=CARTESIAN_POINT('Origin',(4.572,19.748,400.));
#127611=CARTESIAN_POINT('',(-2.477,19.939,400.));
#127612=CARTESIAN_POINT('Origin',(0.,19.4945,400.));
#127613=CARTESIAN_POINT('',(-4.954,19.939,400.));
#127614=CARTESIAN_POINT('',(-4.954,14.858,400.));
#127615=CARTESIAN_POINT('',(-4.954,17.17625,400.));
#127616=CARTESIAN_POINT('',(-4.572,19.939,400.));
#127617=CARTESIAN_POINT('',(-2.477,19.939,400.));
#127618=CARTESIAN_POINT('',(-4.763,19.748,400.));
#127619=CARTESIAN_POINT('Origin',(-4.572,19.748,400.));
#127620=CARTESIAN_POINT('',(-4.763,15.049,400.));
#127621=CARTESIAN_POINT('',(-4.763,19.748,400.));
#127622=CARTESIAN_POINT('Origin',(-4.954,15.049,400.));
#127623=CARTESIAN_POINT('Origin',(4.572,19.748,400.));
#127624=CARTESIAN_POINT('',(4.763,19.748,400.));
#127625=CARTESIAN_POINT('',(4.572,19.939,400.));
#127626=CARTESIAN_POINT('Origin',(4.763,15.049,400.));
#127627=CARTESIAN_POINT('',(4.763,15.049,400.));
#127628=CARTESIAN_POINT('Origin',(4.954,15.049,400.));
#127629=CARTESIAN_POINT('',(4.954,14.858,400.));
#127630=CARTESIAN_POINT('Origin',(7.291,22.736,400.));
#127631=CARTESIAN_POINT('Origin',(-7.291,22.736,400.));
#127632=CARTESIAN_POINT('Origin',(-4.954,15.049,400.));
#127633=CARTESIAN_POINT('',(-4.763,15.049,400.));
#127634=CARTESIAN_POINT('',(-4.954,14.858,400.));
#127635=CARTESIAN_POINT('Origin',(-4.763,19.748,400.));
#127636=CARTESIAN_POINT('',(-4.763,19.748,400.));
#127637=CARTESIAN_POINT('Origin',(-4.572,19.748,400.));
#127638=CARTESIAN_POINT('',(-4.572,19.939,400.));
#127639=CARTESIAN_POINT('Origin',(0.,17.2745,4.));
#127640=CARTESIAN_POINT('',(-6.81246236636335,15.2682931400241,4.));
#127641=CARTESIAN_POINT('',(-6.80496662630522,14.858,4.));
#127642=CARTESIAN_POINT('',(-6.87343118006261,18.6055334688258,4.));
#127643=CARTESIAN_POINT('',(-6.89783581472438,14.858,4.));
#127644=CARTESIAN_POINT('Origin',(-10.752,15.874,4.));
#127645=CARTESIAN_POINT('',(-2.477,14.858,4.));
#127646=CARTESIAN_POINT('Origin',(0.,17.2745,4.));
#127647=CARTESIAN_POINT('',(6.9,14.858,4.));
#127648=CARTESIAN_POINT('',(6.9000000000081,16.898174578473,4.));
#127649=CARTESIAN_POINT('',(6.9,16.06625,4.));
#127650=CARTESIAN_POINT('',(6.89783581472438,14.858,4.));
#127651=CARTESIAN_POINT('',(-2.477,14.858,4.));
#127652=CARTESIAN_POINT('Origin',(10.752,15.874,4.));
#127653=CARTESIAN_POINT('Origin',(0.,17.2745,4.));
#127654=CARTESIAN_POINT('',(-6.83721545938402,16.6231992843132,4.));
#127655=CARTESIAN_POINT('Origin',(-10.752,15.874,4.));
#127656=CARTESIAN_POINT('',(-6.87343118006261,18.6055334688258,4.));
#127657=CARTESIAN_POINT('Origin',(6.9,14.858,0.));
#127658=CARTESIAN_POINT('',(6.9000000000081,16.898174578473,0.));
#127659=CARTESIAN_POINT('',(6.9,16.89817457841,-22.));
#127660=CARTESIAN_POINT('',(6.9,20.058,0.));
#127661=CARTESIAN_POINT('',(6.9,17.17625,0.));
#127662=CARTESIAN_POINT('',(6.9,20.058,0.));
#127663=CARTESIAN_POINT('',(6.9,14.858,0.));
#127664=CARTESIAN_POINT('Origin',(-8.847,15.049,0.));
#127665=CARTESIAN_POINT('',(-8.847,19.4868506020415,0.));
#127666=CARTESIAN_POINT('',(-8.847,19.4868506020415,-22.));
#127667=CARTESIAN_POINT('',(-8.847,19.4868506020415,-16.));
#127668=CARTESIAN_POINT('',(-8.847,22.145,0.));
#127669=CARTESIAN_POINT('',(-8.847,17.27175,0.));
#127670=CARTESIAN_POINT('',(-8.847,22.145,-22.));
#127671=CARTESIAN_POINT('',(-8.847,22.145,0.));
#127672=CARTESIAN_POINT('',(-8.847,17.27175,-22.));
#127673=CARTESIAN_POINT('Origin',(0.,19.4945,0.));
#127674=CARTESIAN_POINT('',(8.751846859637,19.321640494912,0.));
#127675=CARTESIAN_POINT('Origin',(10.752,15.874,0.));
#127676=CARTESIAN_POINT('',(8.847,19.4868506020415,0.));
#127677=CARTESIAN_POINT('Origin',(8.656,19.4868506020415,0.));
#127678=CARTESIAN_POINT('',(8.847,22.145,0.));
#127679=CARTESIAN_POINT('',(8.847,20.92425,0.));
#127680=CARTESIAN_POINT('',(7.291,22.145,0.));
#127681=CARTESIAN_POINT('',(3.6455,22.145,0.));
#127682=CARTESIAN_POINT('',(6.7,22.736,0.));
#127683=CARTESIAN_POINT('Origin',(7.291,22.736,0.));
#127684=CARTESIAN_POINT('',(6.7,23.731,0.));
#127685=CARTESIAN_POINT('',(6.7,21.71725,0.));
#127686=CARTESIAN_POINT('',(-6.7,23.731,0.));
#127687=CARTESIAN_POINT('',(-3.4545,23.731,0.));
#127688=CARTESIAN_POINT('',(-6.7,22.736,0.));
#127689=CARTESIAN_POINT('',(-6.7,21.11525,0.));
#127690=CARTESIAN_POINT('',(-7.291,22.145,0.));
#127691=CARTESIAN_POINT('Origin',(-7.291,22.736,0.));
#127692=CARTESIAN_POINT('',(-4.528,22.145,0.));
#127693=CARTESIAN_POINT('',(-8.751846859637,19.321640494912,0.));
#127694=CARTESIAN_POINT('Origin',(-8.656,19.4868506020415,0.));
#127695=CARTESIAN_POINT('',(-6.83721545938402,16.6231992843132,0.));
#127696=CARTESIAN_POINT('Origin',(-10.752,15.874,0.));
#127697=CARTESIAN_POINT('',(-6.89996662630522,20.058,0.));
#127698=CARTESIAN_POINT('',(-6.89370326010986,19.7151631135172,0.));
#127699=CARTESIAN_POINT('',(3.55,20.058,0.));
#127700=CARTESIAN_POINT('Origin',(-6.90003336812669,20.0616532365438,0.));
#127701=CARTESIAN_POINT('',(-6.83721545938402,16.6231992843132,-22.));
#127702=CARTESIAN_POINT('',(-6.80496662630522,14.858,0.));
#127703=CARTESIAN_POINT('',(-6.89996662630522,20.058,0.));
#127704=CARTESIAN_POINT('Origin',(8.656,19.4868506020415,-22.));
#127705=CARTESIAN_POINT('',(8.751846859637,19.321640494912,-22.));
#127706=CARTESIAN_POINT('',(8.847,19.4868506020415,-22.));
#127707=CARTESIAN_POINT('Origin',(8.656,19.4868506020415,-22.));
#127708=CARTESIAN_POINT('',(8.847,19.4868506020415,-16.));
#127709=CARTESIAN_POINT('',(8.751846859637,19.321640494912,-16.));
#127710=CARTESIAN_POINT('Origin',(8.847,22.354,0.));
#127711=CARTESIAN_POINT('',(8.847,22.145,-22.));
#127712=CARTESIAN_POINT('',(8.847,20.92425,-22.));
#127713=CARTESIAN_POINT('',(8.847,22.145,0.));
#127714=CARTESIAN_POINT('Origin',(0.,19.4945,-22.));
#127715=CARTESIAN_POINT('',(6.89783581472438,14.858,-22.));
#127716=CARTESIAN_POINT('Origin',(10.752,15.874,-22.));
#127717=CARTESIAN_POINT('',(4.954,14.858,-22.));
#127718=CARTESIAN_POINT('',(4.954,14.858,-22.));
#127719=CARTESIAN_POINT('',(4.763,15.049,-22.));
#127720=CARTESIAN_POINT('Origin',(4.954,15.049,-22.));
#127721=CARTESIAN_POINT('',(4.763,19.748,-22.));
#127722=CARTESIAN_POINT('',(4.763,19.748,-22.));
#127723=CARTESIAN_POINT('',(4.572,19.939,-22.));
#127724=CARTESIAN_POINT('Origin',(4.572,19.748,-22.));
#127725=CARTESIAN_POINT('',(-4.572,19.939,-22.));
#127726=CARTESIAN_POINT('',(-4.572,19.939,-22.));
#127727=CARTESIAN_POINT('',(-4.763,19.748,-22.));
#127728=CARTESIAN_POINT('Origin',(-4.572,19.748,-22.));
#127729=CARTESIAN_POINT('',(-4.763,15.049,-22.));
#127730=CARTESIAN_POINT('',(-4.763,19.748,-22.));
#127731=CARTESIAN_POINT('',(-4.954,14.858,-22.));
#127732=CARTESIAN_POINT('Origin',(-4.954,15.049,-22.));
#127733=CARTESIAN_POINT('',(-6.89783581472438,14.858,-22.));
#127734=CARTESIAN_POINT('',(-6.898,14.858,-22.));
#127735=CARTESIAN_POINT('',(-8.751846859637,19.321640494912,-22.));
#127736=CARTESIAN_POINT('Origin',(-10.752,15.874,-22.));
#127737=CARTESIAN_POINT('Origin',(-8.656,19.4868506020415,-22.));
#127738=CARTESIAN_POINT('',(-7.291,22.145,-22.));
#127739=CARTESIAN_POINT('',(-4.528,22.145,-22.));
#127740=CARTESIAN_POINT('',(-6.7,22.736,-22.));
#127741=CARTESIAN_POINT('Origin',(-7.291,22.736,-22.));
#127742=CARTESIAN_POINT('',(-6.7,23.731,-22.));
#127743=CARTESIAN_POINT('',(-6.7,21.11525,-22.));
#127744=CARTESIAN_POINT('',(6.7,23.731,-22.));
#127745=CARTESIAN_POINT('',(-3.4545,23.731,-22.));
#127746=CARTESIAN_POINT('',(6.7,22.736,-22.));
#127747=CARTESIAN_POINT('',(6.7,21.71725,-22.));
#127748=CARTESIAN_POINT('',(7.291,22.145,-22.));
#127749=CARTESIAN_POINT('Origin',(7.291,22.736,-22.));
#127750=CARTESIAN_POINT('',(3.6455,22.145,-22.));
#127751=CARTESIAN_POINT('Origin',(-4.954,14.858,0.));
#127752=CARTESIAN_POINT('',(4.954,14.858,0.));
#127753=CARTESIAN_POINT('',(4.954,14.858,0.));
#127754=CARTESIAN_POINT('',(4.954,14.858,0.));
#127755=CARTESIAN_POINT('',(6.89783581472438,14.858,-22.));
#127756=CARTESIAN_POINT('Origin',(-8.656,19.4868506020415,-22.));
#127757=CARTESIAN_POINT('',(-8.751846859637,19.321640494912,-22.));
#127758=CARTESIAN_POINT('Origin',(7.291,22.145,0.));
#127759=CARTESIAN_POINT('',(7.291,22.145,0.));
#127760=CARTESIAN_POINT('Origin',(-6.909,23.731,0.));
#127761=CARTESIAN_POINT('',(-6.7,23.731,0.));
#127762=CARTESIAN_POINT('',(6.7,23.731,0.));
#127763=CARTESIAN_POINT('',(6.109,23.731,-0.8));
#127764=CARTESIAN_POINT('',(-6.109,23.731,-0.800000000000001));
#127765=CARTESIAN_POINT('',(-0.399999999999999,23.731,-0.8));
#127766=CARTESIAN_POINT('',(-6.109,23.731,-21.2));
#127767=CARTESIAN_POINT('',(-6.109,23.731,-0.4));
#127768=CARTESIAN_POINT('',(6.109,23.731,-21.2));
#127769=CARTESIAN_POINT('',(-6.509,23.731,-21.2));
#127770=CARTESIAN_POINT('',(6.109,23.731,-10.6));
#127771=CARTESIAN_POINT('Origin',(6.7,23.94,0.));
#127772=CARTESIAN_POINT('',(6.7,22.736,0.));
#127773=CARTESIAN_POINT('Origin',(-6.7,22.736,0.));
#127774=CARTESIAN_POINT('',(-6.7,22.736,0.));
#127775=CARTESIAN_POINT('Origin',(-9.056,22.145,0.));
#127776=CARTESIAN_POINT('',(-7.291,22.145,0.));
#127777=CARTESIAN_POINT('Origin',(10.752,15.874,-22.));
#127778=CARTESIAN_POINT('Origin',(-10.752,15.874,-22.));
#127779=CARTESIAN_POINT('',(-6.89783581472438,14.858,-22.));
#127780=CARTESIAN_POINT('Origin',(6.109,24.131,-0.8));
#127781=CARTESIAN_POINT('',(6.109,23.931,-0.800000000000001));
#127782=CARTESIAN_POINT('',(6.109,24.131,-0.8));
#127783=CARTESIAN_POINT('',(-6.109,23.931,-0.800000000000001));
#127784=CARTESIAN_POINT('',(-6.109,23.931,-0.8));
#127785=CARTESIAN_POINT('',(-6.109,24.131,-0.800000000000001));
#127786=CARTESIAN_POINT('Origin',(6.109,24.131,-21.2));
#127787=CARTESIAN_POINT('',(6.109,23.931,-21.2));
#127788=CARTESIAN_POINT('',(6.109,24.131,-21.2));
#127789=CARTESIAN_POINT('',(6.109,23.931,-0.8));
#127790=CARTESIAN_POINT('Origin',(-6.109,24.131,-21.2));
#127791=CARTESIAN_POINT('',(-6.109,23.931,-21.2));
#127792=CARTESIAN_POINT('',(-6.109,24.131,-21.2));
#127793=CARTESIAN_POINT('',(6.109,23.931,-21.2));
#127794=CARTESIAN_POINT('Origin',(-6.109,24.131,-0.800000000000001));
#127795=CARTESIAN_POINT('',(-6.109,23.931,-21.2));
#127796=CARTESIAN_POINT('Origin',(1.11022302462516E-15,23.931,-11.));
#127797=CARTESIAN_POINT('Origin',(7.1,20.058,0.));
#127798=CARTESIAN_POINT('Origin',(4.954,17.858,0.));
#127799=CARTESIAN_POINT('',(4.954,19.939,0.));
#127800=CARTESIAN_POINT('',(4.954,18.67625,0.));
#127801=CARTESIAN_POINT('',(4.954,19.939,0.));
#127802=CARTESIAN_POINT('Origin',(-4.954,14.858,0.));
#127803=CARTESIAN_POINT('',(-4.954,19.939,0.));
#127804=CARTESIAN_POINT('',(-4.954,14.858,0.));
#127805=CARTESIAN_POINT('',(-4.954,17.17625,0.));
#127806=CARTESIAN_POINT('',(-4.954,19.939,400.));
#127807=CARTESIAN_POINT('',(-4.954,14.858,0.));
#127808=CARTESIAN_POINT('Origin',(0.,19.4945,0.));
#127809=CARTESIAN_POINT('',(4.572,19.939,0.));
#127810=CARTESIAN_POINT('',(-2.477,19.939,0.));
#127811=CARTESIAN_POINT('',(4.763,19.748,0.));
#127812=CARTESIAN_POINT('Origin',(4.572,19.748,0.));
#127813=CARTESIAN_POINT('',(4.763,15.049,0.));
#127814=CARTESIAN_POINT('',(4.763,19.748,0.));
#127815=CARTESIAN_POINT('Origin',(4.954,15.049,0.));
#127816=CARTESIAN_POINT('Origin',(0.,19.4945,0.));
#127817=CARTESIAN_POINT('',(-4.763,15.049,0.));
#127818=CARTESIAN_POINT('Origin',(-4.954,15.049,0.));
#127819=CARTESIAN_POINT('',(-4.763,19.748,0.));
#127820=CARTESIAN_POINT('',(-4.763,19.748,0.));
#127821=CARTESIAN_POINT('',(-4.572,19.939,0.));
#127822=CARTESIAN_POINT('Origin',(-4.572,19.748,0.));
#127823=CARTESIAN_POINT('',(-2.477,19.939,0.));
#127824=CARTESIAN_POINT('Origin',(-4.954,14.858,0.));
#127825=CARTESIAN_POINT('',(-4.954,14.858,0.));
#127826=CARTESIAN_POINT('Origin',(4.572,19.939,0.));
#127827=CARTESIAN_POINT('',(-4.572,19.939,0.));
#127828=CARTESIAN_POINT('',(4.572,19.939,0.));
#127829=CARTESIAN_POINT('Origin',(4.572,19.748,0.));
#127830=CARTESIAN_POINT('',(4.763,19.748,0.));
#127831=CARTESIAN_POINT('Origin',(4.763,15.049,0.));
#127832=CARTESIAN_POINT('',(4.763,15.049,0.));
#127833=CARTESIAN_POINT('Origin',(4.954,15.049,0.));
#127834=CARTESIAN_POINT('Origin',(7.291,22.736,0.));
#127835=CARTESIAN_POINT('Origin',(-7.291,22.736,0.));
#127836=CARTESIAN_POINT('Origin',(-4.954,15.049,0.));
#127837=CARTESIAN_POINT('',(-4.763,15.049,0.));
#127838=CARTESIAN_POINT('Origin',(-4.763,19.748,0.));
#127839=CARTESIAN_POINT('',(-4.763,19.748,0.));
#127840=CARTESIAN_POINT('Origin',(-4.572,19.748,0.));
#215595=UNCERTAINTY_MEASURE_WITH_UNIT(LENGTH_MEASURE(0.01),#215610,
'DISTANCE_ACCURACY_VALUE',
'Maximum model space distance between geometric entities at asserted c
onnectivities');
#215598=UNCERTAINTY_MEASURE_WITH_UNIT(LENGTH_MEASURE(0.01),#215610,
'DISTANCE_ACCURACY_VALUE',
'Maximum model space distance between geometric entities at asserted c
onnectivities');
#215606=(
GEOMETRIC_REPRESENTATION_CONTEXT(3)
GLOBAL_UNCERTAINTY_ASSIGNED_CONTEXT((#215595))
GLOBAL_UNIT_ASSIGNED_CONTEXT((#215610,#215612,#215613))
REPRESENTATION_CONTEXT('','3D')
);
#215609=(
GEOMETRIC_REPRESENTATION_CONTEXT(3)
GLOBAL_UNCERTAINTY_ASSIGNED_CONTEXT((#215598))
GLOBAL_UNIT_ASSIGNED_CONTEXT((#215610,#215612,#215613))
REPRESENTATION_CONTEXT('','3D')
);
#215610=(
LENGTH_UNIT()
NAMED_UNIT(*)
SI_UNIT(.MILLI.,.METRE.)
);
#215612=(
NAMED_UNIT(*)
PLANE_ANGLE_UNIT()
SI_UNIT($,.RADIAN.)
);
#215613=(
NAMED_UNIT(*)
SI_UNIT($,.STERADIAN.)
SOLID_ANGLE_UNIT()
);
#215621=SHAPE_DEFINITION_REPRESENTATION(#215633,#215650);
#215633=PRODUCT_DEFINITION_SHAPE('',$,#215661);
#215650=SHAPE_REPRESENTATION('',(#29433),#215606);
#215653=PRODUCT_DEFINITION_CONTEXT('part definition',#215685,'design');
#215661=PRODUCT_DEFINITION('2026-10-04-16-15-13-894','Carriage_Base',#215671,
#215653);
#215671=PRODUCT_DEFINITION_FORMATION('',$,#215694);
#215685=APPLICATION_CONTEXT(
'Core Data for Automotive Mechanical Design Process');
#215686=PRODUCT_CONTEXT('part definition',#215685,'mechanical');
#215694=PRODUCT('2026-10-04-16-15-13-894','Carriage_Base',$,(#215686));
#215698=PRESENTATION_STYLE_ASSIGNMENT((#215700));
#215700=SURFACE_STYLE_USAGE(.BOTH.,#215702);
#215702=SURFACE_SIDE_STYLE('',(#215704));
#215704=SURFACE_STYLE_FILL_AREA(#215706);
#215706=FILL_AREA_STYLE('Opaque(245,245,246)',(#215708));
#215708=FILL_AREA_STYLE_COLOUR('Opaque(245,245,246)',#215710);
#215710=COLOUR_RGB('Opaque(245,245,246)', 0.66274510, 0.83137255, 0.94901961);
ENDSEC;
END-ISO-10303-21;
